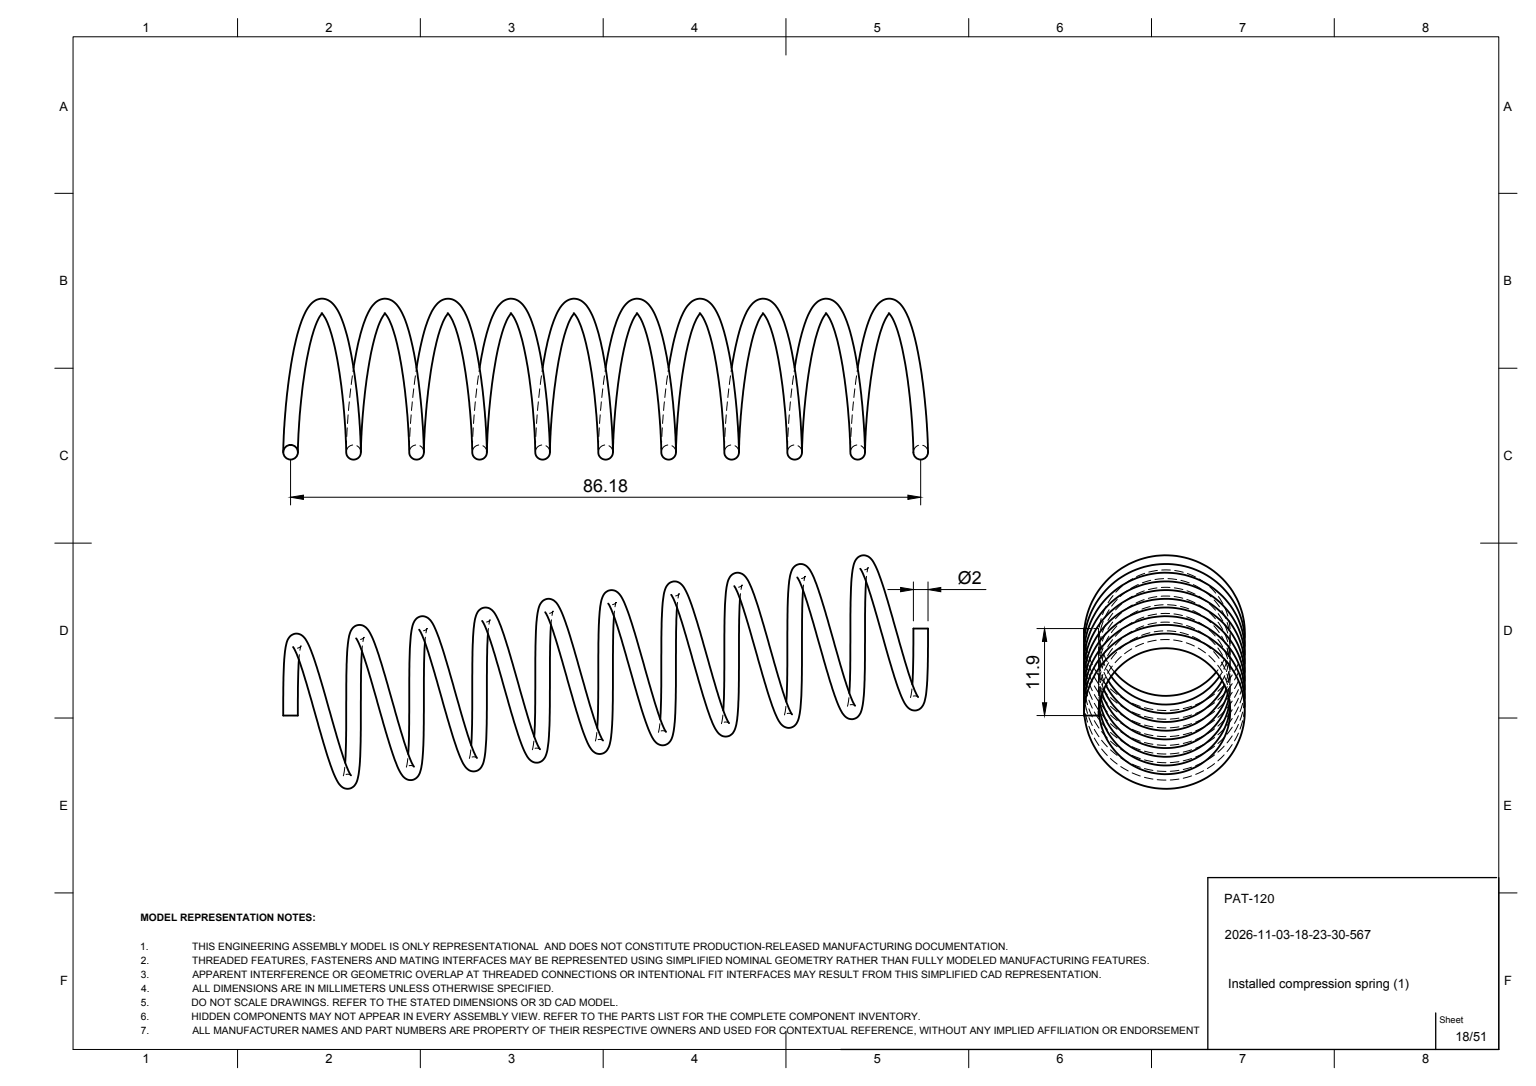
ISO-10303-21;
HEADER;
/* Generated by software containing ST-Developer
 * from STEP Tools, Inc. (www.steptools.com) 
 */

FILE_DESCRIPTION(
/* description */ ('Vibration shaker table dummy'),
/* implementation_level */ '2;1');

FILE_NAME(
/* name */ 'Installed compression spring (1).step',
/* time_stamp */ '2026-10-27T10:55:14-07:00',
/* author */ (''),
/* organization */ (''),
/* preprocessor_version */ 'ST-DEVELOPER v20.2',
/* originating_system */ 'Autodesk Translation Framework v15.17.0.0',
/* authorisation */ '');

FILE_SCHEMA (('AUTOMOTIVE_DESIGN { 1 0 10303 214 3 1 1 }'));
ENDSEC;

DATA;
#10=MECHANICAL_DESIGN_GEOMETRIC_PRESENTATION_REPRESENTATION('',(#699),#22394);
#587=B_SPLINE_CURVE_WITH_KNOTS('',3,(#17470,#17471,#17472,#17473,#17474,
#17475,#17476,#17477,#17478,#17479,#17480,#17481,#17482,#17483,#17484,#17485,
#17486,#17487,#17488,#17489,#17490,#17491,#17492,#17493,#17494,#17495,#17496,
#17497,#17498,#17499,#17500,#17501,#17502,#17503,#17504,#17505,#17506,#17507,
#17508,#17509,#17510,#17511,#17512,#17513,#17514,#17515,#17516,#17517,#17518,
#17519,#17520,#17521,#17522,#17523,#17524,#17525,#17526,#17527,#17528,#17529,
#17530,#17531,#17532,#17533,#17534,#17535,#17536,#17537,#17538,#17539,#17540,
#17541,#17542,#17543,#17544,#17545,#17546,#17547,#17548,#17549,#17550,#17551,
#17552,#17553,#17554,#17555,#17556,#17557,#17558,#17559,#17560,#17561,#17562,
#17563,#17564,#17565,#17566,#17567,#17568,#17569,#17570,#17571,#17572,#17573,
#17574,#17575,#17576,#17577,#17578,#17579,#17580,#17581,#17582,#17583,#17584,
#17585,#17586,#17587,#17588,#17589,#17590,#17591,#17592,#17593,#17594,#17595,
#17596),.UNSPECIFIED.,.F.,.F.,(4,1,1,1,1,1,1,1,1,1,1,1,1,1,1,1,1,1,1,1,
1,1,1,1,1,1,1,1,1,1,1,1,1,1,1,1,1,1,1,1,1,1,1,1,1,1,1,1,1,1,1,1,1,1,1,1,
1,1,1,1,1,1,1,1,1,1,1,1,1,1,1,1,1,1,1,1,1,1,1,1,1,1,1,1,1,1,1,1,1,1,1,1,
1,1,1,1,1,1,1,1,1,1,1,1,1,1,1,1,1,1,1,1,1,1,1,1,1,1,1,1,1,1,1,1,4),(0.,
0.00892857142857143,0.0178571428571429,0.0267857142857143,0.0357142857142857,
0.0446428571428571,0.0535714285714286,0.0625,0.0714285714285714,0.0803571428571428,
0.0892857142857143,0.0982142857142857,0.107142857142857,0.116071428571429,
0.125,0.133928571428571,0.142857142857143,0.150793650793651,0.158730158730159,
0.166666666666667,0.174603174603175,0.182539682539683,0.19047619047619,
0.196428571428571,0.202380952380952,0.208333333333333,0.214285714285714,
0.222222222222222,0.23015873015873,0.238095238095238,0.244047619047619,
0.25,0.261904761904762,0.273809523809524,0.285714285714286,0.297619047619048,
0.30952380952381,0.321428571428571,0.333333333333333,0.337301587301587,
0.341269841269841,0.349206349206349,0.357142857142857,0.365079365079365,
0.373015873015873,0.380952380952381,0.386904761904762,0.392857142857143,
0.404761904761905,0.410714285714286,0.416666666666667,0.422619047619048,
0.428571428571429,0.4375,0.446428571428571,0.455357142857143,0.459821428571429,
0.464285714285714,0.470238095238095,0.476190476190476,0.482142857142857,
0.491071428571429,0.5,0.508928571428571,0.517857142857143,0.526785714285714,
0.535714285714286,0.544642857142857,0.553571428571429,0.5625,0.571428571428571,
0.580357142857143,0.589285714285714,0.598214285714286,0.607142857142857,
0.616071428571429,0.625,0.633928571428571,0.642857142857143,0.650793650793651,
0.658730158730159,0.666666666666667,0.672619047619048,0.678571428571428,
0.684523809523809,0.69047619047619,0.696428571428571,0.702380952380952,
0.708333333333333,0.714285714285714,0.720238095238095,0.726190476190476,
0.732142857142857,0.738095238095238,0.744047619047619,0.75,0.755952380952381,
0.761904761904762,0.76984126984127,0.777777777777778,0.785714285714286,
0.794642857142857,0.803571428571428,0.8125,0.821428571428571,0.830357142857143,
0.839285714285714,0.848214285714286,0.857142857142857,0.866071428571429,
0.875,0.883928571428571,0.892857142857143,0.901785714285714,0.910714285714286,
0.919642857142857,0.928571428571429,0.9375,0.946428571428571,0.955357142857143,
0.964285714285714,0.973214285714286,0.982142857142857,0.991071428571429,
1.),.UNSPECIFIED.);
#591=B_SPLINE_SURFACE_WITH_KNOTS('',3,3,((#16197,#16198,#16199,#16200,#16201,
#16202,#16203,#16204,#16205,#16206,#16207,#16208,#16209,#16210,#16211,#16212,
#16213,#16214,#16215,#16216,#16217,#16218,#16219,#16220,#16221,#16222,#16223,
#16224,#16225,#16226,#16227,#16228,#16229,#16230,#16231,#16232,#16233,#16234,
#16235,#16236,#16237,#16238,#16239,#16240,#16241,#16242,#16243,#16244,#16245,
#16246,#16247,#16248,#16249,#16250,#16251,#16252,#16253,#16254,#16255,#16256,
#16257,#16258,#16259,#16260,#16261,#16262,#16263,#16264,#16265,#16266,#16267,
#16268,#16269,#16270,#16271,#16272,#16273,#16274,#16275,#16276,#16277,#16278,
#16279,#16280,#16281,#16282,#16283,#16284,#16285,#16286,#16287,#16288,#16289,
#16290,#16291,#16292,#16293,#16294,#16295,#16296,#16297,#16298,#16299,#16300,
#16301,#16302,#16303,#16304,#16305,#16306,#16307,#16308,#16309,#16310,#16311,
#16312,#16313,#16314,#16315,#16316,#16317,#16318,#16319,#16320,#16321,#16322,
#16323),(#16324,#16325,#16326,#16327,#16328,#16329,#16330,#16331,#16332,
#16333,#16334,#16335,#16336,#16337,#16338,#16339,#16340,#16341,#16342,#16343,
#16344,#16345,#16346,#16347,#16348,#16349,#16350,#16351,#16352,#16353,#16354,
#16355,#16356,#16357,#16358,#16359,#16360,#16361,#16362,#16363,#16364,#16365,
#16366,#16367,#16368,#16369,#16370,#16371,#16372,#16373,#16374,#16375,#16376,
#16377,#16378,#16379,#16380,#16381,#16382,#16383,#16384,#16385,#16386,#16387,
#16388,#16389,#16390,#16391,#16392,#16393,#16394,#16395,#16396,#16397,#16398,
#16399,#16400,#16401,#16402,#16403,#16404,#16405,#16406,#16407,#16408,#16409,
#16410,#16411,#16412,#16413,#16414,#16415,#16416,#16417,#16418,#16419,#16420,
#16421,#16422,#16423,#16424,#16425,#16426,#16427,#16428,#16429,#16430,#16431,
#16432,#16433,#16434,#16435,#16436,#16437,#16438,#16439,#16440,#16441,#16442,
#16443,#16444,#16445,#16446,#16447,#16448,#16449,#16450),(#16451,#16452,
#16453,#16454,#16455,#16456,#16457,#16458,#16459,#16460,#16461,#16462,#16463,
#16464,#16465,#16466,#16467,#16468,#16469,#16470,#16471,#16472,#16473,#16474,
#16475,#16476,#16477,#16478,#16479,#16480,#16481,#16482,#16483,#16484,#16485,
#16486,#16487,#16488,#16489,#16490,#16491,#16492,#16493,#16494,#16495,#16496,
#16497,#16498,#16499,#16500,#16501,#16502,#16503,#16504,#16505,#16506,#16507,
#16508,#16509,#16510,#16511,#16512,#16513,#16514,#16515,#16516,#16517,#16518,
#16519,#16520,#16521,#16522,#16523,#16524,#16525,#16526,#16527,#16528,#16529,
#16530,#16531,#16532,#16533,#16534,#16535,#16536,#16537,#16538,#16539,#16540,
#16541,#16542,#16543,#16544,#16545,#16546,#16547,#16548,#16549,#16550,#16551,
#16552,#16553,#16554,#16555,#16556,#16557,#16558,#16559,#16560,#16561,#16562,
#16563,#16564,#16565,#16566,#16567,#16568,#16569,#16570,#16571,#16572,#16573,
#16574,#16575,#16576,#16577),(#16578,#16579,#16580,#16581,#16582,#16583,
#16584,#16585,#16586,#16587,#16588,#16589,#16590,#16591,#16592,#16593,#16594,
#16595,#16596,#16597,#16598,#16599,#16600,#16601,#16602,#16603,#16604,#16605,
#16606,#16607,#16608,#16609,#16610,#16611,#16612,#16613,#16614,#16615,#16616,
#16617,#16618,#16619,#16620,#16621,#16622,#16623,#16624,#16625,#16626,#16627,
#16628,#16629,#16630,#16631,#16632,#16633,#16634,#16635,#16636,#16637,#16638,
#16639,#16640,#16641,#16642,#16643,#16644,#16645,#16646,#16647,#16648,#16649,
#16650,#16651,#16652,#16653,#16654,#16655,#16656,#16657,#16658,#16659,#16660,
#16661,#16662,#16663,#16664,#16665,#16666,#16667,#16668,#16669,#16670,#16671,
#16672,#16673,#16674,#16675,#16676,#16677,#16678,#16679,#16680,#16681,#16682,
#16683,#16684,#16685,#16686,#16687,#16688,#16689,#16690,#16691,#16692,#16693,
#16694,#16695,#16696,#16697,#16698,#16699,#16700,#16701,#16702,#16703,#16704),
(#16705,#16706,#16707,#16708,#16709,#16710,#16711,#16712,#16713,#16714,
#16715,#16716,#16717,#16718,#16719,#16720,#16721,#16722,#16723,#16724,#16725,
#16726,#16727,#16728,#16729,#16730,#16731,#16732,#16733,#16734,#16735,#16736,
#16737,#16738,#16739,#16740,#16741,#16742,#16743,#16744,#16745,#16746,#16747,
#16748,#16749,#16750,#16751,#16752,#16753,#16754,#16755,#16756,#16757,#16758,
#16759,#16760,#16761,#16762,#16763,#16764,#16765,#16766,#16767,#16768,#16769,
#16770,#16771,#16772,#16773,#16774,#16775,#16776,#16777,#16778,#16779,#16780,
#16781,#16782,#16783,#16784,#16785,#16786,#16787,#16788,#16789,#16790,#16791,
#16792,#16793,#16794,#16795,#16796,#16797,#16798,#16799,#16800,#16801,#16802,
#16803,#16804,#16805,#16806,#16807,#16808,#16809,#16810,#16811,#16812,#16813,
#16814,#16815,#16816,#16817,#16818,#16819,#16820,#16821,#16822,#16823,#16824,
#16825,#16826,#16827,#16828,#16829,#16830,#16831),(#16832,#16833,#16834,
#16835,#16836,#16837,#16838,#16839,#16840,#16841,#16842,#16843,#16844,#16845,
#16846,#16847,#16848,#16849,#16850,#16851,#16852,#16853,#16854,#16855,#16856,
#16857,#16858,#16859,#16860,#16861,#16862,#16863,#16864,#16865,#16866,#16867,
#16868,#16869,#16870,#16871,#16872,#16873,#16874,#16875,#16876,#16877,#16878,
#16879,#16880,#16881,#16882,#16883,#16884,#16885,#16886,#16887,#16888,#16889,
#16890,#16891,#16892,#16893,#16894,#16895,#16896,#16897,#16898,#16899,#16900,
#16901,#16902,#16903,#16904,#16905,#16906,#16907,#16908,#16909,#16910,#16911,
#16912,#16913,#16914,#16915,#16916,#16917,#16918,#16919,#16920,#16921,#16922,
#16923,#16924,#16925,#16926,#16927,#16928,#16929,#16930,#16931,#16932,#16933,
#16934,#16935,#16936,#16937,#16938,#16939,#16940,#16941,#16942,#16943,#16944,
#16945,#16946,#16947,#16948,#16949,#16950,#16951,#16952,#16953,#16954,#16955,
#16956,#16957,#16958),(#16959,#16960,#16961,#16962,#16963,#16964,#16965,
#16966,#16967,#16968,#16969,#16970,#16971,#16972,#16973,#16974,#16975,#16976,
#16977,#16978,#16979,#16980,#16981,#16982,#16983,#16984,#16985,#16986,#16987,
#16988,#16989,#16990,#16991,#16992,#16993,#16994,#16995,#16996,#16997,#16998,
#16999,#17000,#17001,#17002,#17003,#17004,#17005,#17006,#17007,#17008,#17009,
#17010,#17011,#17012,#17013,#17014,#17015,#17016,#17017,#17018,#17019,#17020,
#17021,#17022,#17023,#17024,#17025,#17026,#17027,#17028,#17029,#17030,#17031,
#17032,#17033,#17034,#17035,#17036,#17037,#17038,#17039,#17040,#17041,#17042,
#17043,#17044,#17045,#17046,#17047,#17048,#17049,#17050,#17051,#17052,#17053,
#17054,#17055,#17056,#17057,#17058,#17059,#17060,#17061,#17062,#17063,#17064,
#17065,#17066,#17067,#17068,#17069,#17070,#17071,#17072,#17073,#17074,#17075,
#17076,#17077,#17078,#17079,#17080,#17081,#17082,#17083,#17084,#17085),
(#17086,#17087,#17088,#17089,#17090,#17091,#17092,#17093,#17094,#17095,
#17096,#17097,#17098,#17099,#17100,#17101,#17102,#17103,#17104,#17105,#17106,
#17107,#17108,#17109,#17110,#17111,#17112,#17113,#17114,#17115,#17116,#17117,
#17118,#17119,#17120,#17121,#17122,#17123,#17124,#17125,#17126,#17127,#17128,
#17129,#17130,#17131,#17132,#17133,#17134,#17135,#17136,#17137,#17138,#17139,
#17140,#17141,#17142,#17143,#17144,#17145,#17146,#17147,#17148,#17149,#17150,
#17151,#17152,#17153,#17154,#17155,#17156,#17157,#17158,#17159,#17160,#17161,
#17162,#17163,#17164,#17165,#17166,#17167,#17168,#17169,#17170,#17171,#17172,
#17173,#17174,#17175,#17176,#17177,#17178,#17179,#17180,#17181,#17182,#17183,
#17184,#17185,#17186,#17187,#17188,#17189,#17190,#17191,#17192,#17193,#17194,
#17195,#17196,#17197,#17198,#17199,#17200,#17201,#17202,#17203,#17204,#17205,
#17206,#17207,#17208,#17209,#17210,#17211,#17212),(#17213,#17214,#17215,
#17216,#17217,#17218,#17219,#17220,#17221,#17222,#17223,#17224,#17225,#17226,
#17227,#17228,#17229,#17230,#17231,#17232,#17233,#17234,#17235,#17236,#17237,
#17238,#17239,#17240,#17241,#17242,#17243,#17244,#17245,#17246,#17247,#17248,
#17249,#17250,#17251,#17252,#17253,#17254,#17255,#17256,#17257,#17258,#17259,
#17260,#17261,#17262,#17263,#17264,#17265,#17266,#17267,#17268,#17269,#17270,
#17271,#17272,#17273,#17274,#17275,#17276,#17277,#17278,#17279,#17280,#17281,
#17282,#17283,#17284,#17285,#17286,#17287,#17288,#17289,#17290,#17291,#17292,
#17293,#17294,#17295,#17296,#17297,#17298,#17299,#17300,#17301,#17302,#17303,
#17304,#17305,#17306,#17307,#17308,#17309,#17310,#17311,#17312,#17313,#17314,
#17315,#17316,#17317,#17318,#17319,#17320,#17321,#17322,#17323,#17324,#17325,
#17326,#17327,#17328,#17329,#17330,#17331,#17332,#17333,#17334,#17335,#17336,
#17337,#17338,#17339),(#17340,#17341,#17342,#17343,#17344,#17345,#17346,
#17347,#17348,#17349,#17350,#17351,#17352,#17353,#17354,#17355,#17356,#17357,
#17358,#17359,#17360,#17361,#17362,#17363,#17364,#17365,#17366,#17367,#17368,
#17369,#17370,#17371,#17372,#17373,#17374,#17375,#17376,#17377,#17378,#17379,
#17380,#17381,#17382,#17383,#17384,#17385,#17386,#17387,#17388,#17389,#17390,
#17391,#17392,#17393,#17394,#17395,#17396,#17397,#17398,#17399,#17400,#17401,
#17402,#17403,#17404,#17405,#17406,#17407,#17408,#17409,#17410,#17411,#17412,
#17413,#17414,#17415,#17416,#17417,#17418,#17419,#17420,#17421,#17422,#17423,
#17424,#17425,#17426,#17427,#17428,#17429,#17430,#17431,#17432,#17433,#17434,
#17435,#17436,#17437,#17438,#17439,#17440,#17441,#17442,#17443,#17444,#17445,
#17446,#17447,#17448,#17449,#17450,#17451,#17452,#17453,#17454,#17455,#17456,
#17457,#17458,#17459,#17460,#17461,#17462,#17463,#17464,#17465,#17466)),
 .UNSPECIFIED.,.T.,.F.,.F.,(4,1,1,1,1,1,1,4),(4,1,1,1,1,1,1,1,1,1,1,1,1,
1,1,1,1,1,1,1,1,1,1,1,1,1,1,1,1,1,1,1,1,1,1,1,1,1,1,1,1,1,1,1,1,1,1,1,1,
1,1,1,1,1,1,1,1,1,1,1,1,1,1,1,1,1,1,1,1,1,1,1,1,1,1,1,1,1,1,1,1,1,1,1,1,
1,1,1,1,1,1,1,1,1,1,1,1,1,1,1,1,1,1,1,1,1,1,1,1,1,1,1,1,1,1,1,1,1,1,1,1,
1,1,1,4),(-3.14159265358979,-2.24399475256414,-1.34639685153848,-0.448798950512828,
0.448798950512828,1.34639685153848,2.24399475256414,3.14159265358979),(0.,
0.00892857142857143,0.0178571428571429,0.0267857142857143,0.0357142857142857,
0.0446428571428571,0.0535714285714286,0.0625,0.0714285714285714,0.0803571428571428,
0.0892857142857143,0.0982142857142857,0.107142857142857,0.116071428571429,
0.125,0.133928571428571,0.142857142857143,0.150793650793651,0.158730158730159,
0.166666666666667,0.174603174603175,0.182539682539683,0.19047619047619,
0.196428571428571,0.202380952380952,0.208333333333333,0.214285714285714,
0.222222222222222,0.23015873015873,0.238095238095238,0.244047619047619,
0.25,0.261904761904762,0.273809523809524,0.285714285714286,0.297619047619048,
0.30952380952381,0.321428571428571,0.333333333333333,0.337301587301587,
0.341269841269841,0.349206349206349,0.357142857142857,0.365079365079365,
0.373015873015873,0.380952380952381,0.386904761904762,0.392857142857143,
0.404761904761905,0.410714285714286,0.416666666666667,0.422619047619048,
0.428571428571429,0.4375,0.446428571428571,0.455357142857143,0.459821428571429,
0.464285714285714,0.470238095238095,0.476190476190476,0.482142857142857,
0.491071428571429,0.5,0.508928571428571,0.517857142857143,0.526785714285714,
0.535714285714286,0.544642857142857,0.553571428571429,0.5625,0.571428571428571,
0.580357142857143,0.589285714285714,0.598214285714286,0.607142857142857,
0.616071428571429,0.625,0.633928571428571,0.642857142857143,0.650793650793651,
0.658730158730159,0.666666666666667,0.672619047619048,0.678571428571428,
0.684523809523809,0.69047619047619,0.696428571428571,0.702380952380952,
0.708333333333333,0.714285714285714,0.720238095238095,0.726190476190476,
0.732142857142857,0.738095238095238,0.744047619047619,0.75,0.755952380952381,
0.761904761904762,0.76984126984127,0.777777777777778,0.785714285714286,
0.794642857142857,0.803571428571428,0.8125,0.821428571428571,0.830357142857143,
0.839285714285714,0.848214285714286,0.857142857142857,0.866071428571429,
0.875,0.883928571428571,0.892857142857143,0.901785714285714,0.910714285714286,
0.919642857142857,0.928571428571429,0.9375,0.946428571428571,0.955357142857143,
0.964285714285714,0.973214285714286,0.982142857142857,0.991071428571429,
1.),.UNSPECIFIED.);
#607=SHAPE_REPRESENTATION_RELATIONSHIP('SRR','None',#22653,#653);
#653=ADVANCED_BREP_SHAPE_REPRESENTATION('',(#745),#22359);
#699=STYLED_ITEM('',(#22961),#745);
#745=MANIFOLD_SOLID_BREP('Body1',#9217);
#1146=PLANE('',#10078);
#1147=PLANE('',#10079);
#1496=FACE_OUTER_BOUND('',#2110,.T.);
#1497=FACE_OUTER_BOUND('',#2111,.T.);
#1498=FACE_OUTER_BOUND('',#2112,.T.);
#2110=EDGE_LOOP('',(#6972,#6973,#6974,#6975));
#2111=EDGE_LOOP('',(#6976));
#2112=EDGE_LOOP('',(#6977));
#4006=CIRCLE('',#10076,0.1);
#4007=CIRCLE('',#10077,0.1);
#4609=VERTEX_POINT('',#17467);
#4610=VERTEX_POINT('',#17469);
#5479=EDGE_CURVE('',#4609,#4609,#4006,.T.);
#5480=EDGE_CURVE('',#4609,#4610,#587,.T.);
#5481=EDGE_CURVE('',#4610,#4610,#4007,.T.);
#6972=ORIENTED_EDGE('',*,*,#5479,.T.);
#6973=ORIENTED_EDGE('',*,*,#5480,.T.);
#6974=ORIENTED_EDGE('',*,*,#5481,.F.);
#6975=ORIENTED_EDGE('',*,*,#5480,.F.);
#6976=ORIENTED_EDGE('',*,*,#5481,.T.);
#6977=ORIENTED_EDGE('',*,*,#5479,.F.);
#8861=ADVANCED_FACE('',(#1496),#591,.T.);
#8862=ADVANCED_FACE('',(#1497),#1146,.T.);
#8863=ADVANCED_FACE('',(#1498),#1147,.F.);
#9217=CLOSED_SHELL('',(#8861,#8862,#8863));
#10075=AXIS2_PLACEMENT_3D('',#16196,#11796,#11797);
#10076=AXIS2_PLACEMENT_3D('',#17468,#11798,#11799);
#10077=AXIS2_PLACEMENT_3D('',#17597,#11800,#11801);
#10078=AXIS2_PLACEMENT_3D('',#17598,#11802,#11803);
#10079=AXIS2_PLACEMENT_3D('',#17599,#11804,#11805);
#11796=DIRECTION('axis',(0.,0.,1.));
#11797=DIRECTION('refdir',(1.,0.,0.));
#11798=DIRECTION('center_axis',(-0.000133356290794322,0.990604928516086,
0.136754735990165));
#11799=DIRECTION('ref_axis',(1.84100680806489E-5,-0.136754734750974,0.990604937492369));
#11800=DIRECTION('center_axis',(0.000133356202123069,0.990604928495684,
0.13675473613804));
#11801=DIRECTION('ref_axis',(-0.722226697925981,0.0946826990341326,-0.685145081939983));
#11802=DIRECTION('center_axis',(0.000133356202123069,0.990604928495684,
0.13675473613804));
#11803=DIRECTION('ref_axis',(-0.722226697925981,0.0946826990341325,-0.685145081939983));
#11804=DIRECTION('center_axis',(-0.000133356290794322,0.990604928516086,
0.136754735990165));
#11805=DIRECTION('ref_axis',(1.84100680806489E-5,-0.136754734750974,0.990604937492369));
#16196=CARTESIAN_POINT('',(0.,0.,0.));
#16197=CARTESIAN_POINT('Ctrl Pts',(-5.00000184100681,4.0136754734751,2.60093950625076));
#16198=CARTESIAN_POINT('Ctrl Pts',(-5.00002711936209,4.20144961727963,2.62686205390075));
#16199=CARTESIAN_POINT('Ctrl Pts',(-5.1076914443916,4.57620101292901,2.67882571929646));
#16200=CARTESIAN_POINT('Ctrl Pts',(-5.54731085839696,4.97011855968613,2.75738770095752));
#16201=CARTESIAN_POINT('Ctrl Pts',(-6.13330829028169,5.07009398433603,2.83651804650349));
#16202=CARTESIAN_POINT('Ctrl Pts',(-6.68676060294283,4.84148936906199,2.91622569034364));
#16203=CARTESIAN_POINT('Ctrl Pts',(-7.03617542740839,4.34995411926946,2.99649057036664));
#16204=CARTESIAN_POINT('Ctrl Pts',(-7.07077171566156,3.74380977688242,3.07730075350998));
#16205=CARTESIAN_POINT('Ctrl Pts',(-6.77566001133407,3.20870450421941,3.15863603264667));
#16206=CARTESIAN_POINT('Ctrl Pts',(-6.23777975703619,2.91082274760045,3.24047540010177));
#16207=CARTESIAN_POINT('Ctrl Pts',(-5.62027751939497,2.94499359194798,3.32279385402167));
#16208=CARTESIAN_POINT('Ctrl Pts',(-5.1128578559771,3.30444603110391,3.40556404882598));
#16209=CARTESIAN_POINT('Ctrl Pts',(-4.87328209631149,3.88170381609706,3.48875576249667));
#16210=CARTESIAN_POINT('Ctrl Pts',(-4.97806047014568,4.50081578134862,3.57233636795591));
#16211=CARTESIAN_POINT('Ctrl Pts',(-5.39799694068156,4.97124635132397,3.65627091939543));
#16212=CARTESIAN_POINT('Ctrl Pts',(-6.00608186722498,5.1467635917961,3.7405223892875));
#16213=CARTESIAN_POINT('Ctrl Pts',(-6.61648592829516,4.97125245378467,3.82505187703477));
#16214=CARTESIAN_POINT('Ctrl Pts',(-7.02504723026834,4.51407458863333,3.90667930466183));
#16215=CARTESIAN_POINT('Ctrl Pts',(-7.14109507248108,3.93953170138583,3.98533819578826));
#16216=CARTESIAN_POINT('Ctrl Pts',(-6.97515546374893,3.40104443225745,4.06097495793453));
#16217=CARTESIAN_POINT('Ctrl Pts',(-6.57122653386479,3.00706128325563,4.13670514732847));
#16218=CARTESIAN_POINT('Ctrl Pts',(-6.02775857632327,2.85377271371871,4.21249751130402));
#16219=CARTESIAN_POINT('Ctrl Pts',(-5.47693199324532,2.97976879840739,4.28832050275612));
#16220=CARTESIAN_POINT('Ctrl Pts',(-5.08889329636147,3.32248782371839,4.35782394322737));
#16221=CARTESIAN_POINT('Ctrl Pts',(-4.90348334427995,3.74815768282725,4.42098503121462));
#16222=CARTESIAN_POINT('Ctrl Pts',(-4.88777846541416,4.16541417756998,4.47779829335302));
#16223=CARTESIAN_POINT('Ctrl Pts',(-5.02572337488508,4.5591407782775,4.53456660974454));
#16224=CARTESIAN_POINT('Ctrl Pts',(-5.32762081329308,4.91046292297288,4.59757802398128));
#16225=CARTESIAN_POINT('Ctrl Pts',(-5.79769987729577,5.12240617534609,4.6667893141555));
#16226=CARTESIAN_POINT('Ctrl Pts',(-6.35744977854988,5.0800953582818,4.74213609062164));
#16227=CARTESIAN_POINT('Ctrl Pts',(-6.7886388886812,4.80135715932747,4.81103357029135));
#16228=CARTESIAN_POINT('Ctrl Pts',(-7.03217914396847,4.41239214657722,4.87351124701705));
#16229=CARTESIAN_POINT('Ctrl Pts',(-7.13592863330475,3.87207852021905,4.94830807653976));
#16230=CARTESIAN_POINT('Ctrl Pts',(-6.87284718079957,3.20107467373212,5.04144479366485));
#16231=CARTESIAN_POINT('Ctrl Pts',(-6.09623481157017,2.82823992504595,5.15254762809713));
#16232=CARTESIAN_POINT('Ctrl Pts',(-5.27971004197149,3.08146490109176,5.26291010705797));
#16233=CARTESIAN_POINT('Ctrl Pts',(-4.85635349881296,3.81715131471987,5.37246078991772));
#16234=CARTESIAN_POINT('Ctrl Pts',(-5.04487949063783,4.63769677411038,5.48113679376609));
#16235=CARTESIAN_POINT('Ctrl Pts',(-5.73589746055469,5.10693196272956,5.58888446285182));
#16236=CARTESIAN_POINT('Ctrl Pts',(-6.37118793757295,5.00949360744693,5.67193196549858));
#16237=CARTESIAN_POINT('Ctrl Pts',(-6.71254361053678,4.74926813559046,5.73087908447486));
#16238=CARTESIAN_POINT('Ctrl Pts',(-6.92618421314144,4.48213635150675,5.77788659686335));
#16239=CARTESIAN_POINT('Ctrl Pts',(-7.05447791083229,4.06557532936466,5.83636209009091));
#16240=CARTESIAN_POINT('Ctrl Pts',(-6.95088091422359,3.55670409484484,5.90607316301112));
#16241=CARTESIAN_POINT('Ctrl Pts',(-6.61900788359635,3.16160526086392,5.97532164754671));
#16242=CARTESIAN_POINT('Ctrl Pts',(-6.14183402203666,2.97493714351951,6.0441065734333));
#16243=CARTESIAN_POINT('Ctrl Pts',(-5.67880942079896,3.03347123408109,6.10673564359386));
#16244=CARTESIAN_POINT('Ctrl Pts',(-5.32735160410172,3.25520230218429,6.16333652454754));
#16245=CARTESIAN_POINT('Ctrl Pts',(-5.03108251682038,3.65479384285351,6.23091649770626));
#16246=CARTESIAN_POINT('Ctrl Pts',(-4.99209121035488,4.17131828916311,6.29799027327816));
#16247=CARTESIAN_POINT('Ctrl Pts',(-5.22308647377139,4.60388582873653,6.36457330678434));
#16248=CARTESIAN_POINT('Ctrl Pts',(-5.49945070307415,4.84205518395227,6.4142703184249));
#16249=CARTESIAN_POINT('Ctrl Pts',(-5.8429108649416,4.96183684549319,6.46373244635463));
#16250=CARTESIAN_POINT('Ctrl Pts',(-6.26484181971828,4.94625056066266,6.52117144061682));
#16251=CARTESIAN_POINT('Ctrl Pts',(-6.69390577408147,4.70907736638303,6.58644589945804));
#16252=CARTESIAN_POINT('Ctrl Pts',(-6.95873462103172,4.22881797506906,6.65940509116432));
#16253=CARTESIAN_POINT('Ctrl Pts',(-6.93269246532923,3.77588585116234,6.71983222414211));
#16254=CARTESIAN_POINT('Ctrl Pts',(-6.77107468324783,3.46412923688142,6.7679659145118));
#16255=CARTESIAN_POINT('Ctrl Pts',(-6.57079871082626,3.25210408080074,6.80796630929164));
#16256=CARTESIAN_POINT('Ctrl Pts',(-6.28566327773964,3.10148204150563,6.85183024182226));
#16257=CARTESIAN_POINT('Ctrl Pts',(-5.9374350403567,3.06238692304077,6.89952195896654));
#16258=CARTESIAN_POINT('Ctrl Pts',(-5.54350254185785,3.16770824417749,6.95498839067594));
#16259=CARTESIAN_POINT('Ctrl Pts',(-5.18977130243312,3.48372162057587,7.01814871426604));
#16260=CARTESIAN_POINT('Ctrl Pts',(-5.04285761799324,3.99497433346206,7.0889328817521));
#16261=CARTESIAN_POINT('Ctrl Pts',(-5.18978309684873,4.50416337482064,7.15948666242575));
#16262=CARTESIAN_POINT('Ctrl Pts',(-5.58408091231752,4.85632154197909,7.22985222665258));
#16263=CARTESIAN_POINT('Ctrl Pts',(-6.10418851591415,4.94454356395432,7.30007283487924));
#16264=CARTESIAN_POINT('Ctrl Pts',(-6.59084588507658,4.74288104801731,7.37019262264957));
#16265=CARTESIAN_POINT('Ctrl Pts',(-6.89540829263521,4.31357351131412,7.44025632549589));
#16266=CARTESIAN_POINT('Ctrl Pts',(-6.92492923689232,3.78812028153619,7.51030900574892));
#16267=CARTESIAN_POINT('Ctrl Pts',(-6.67028427013333,3.32725098620657,7.58039577698737));
#16268=CARTESIAN_POINT('Ctrl Pts',(-6.20897623341015,3.0721729365591,7.65056157443552));
#16269=CARTESIAN_POINT('Ctrl Pts',(-5.68173783558839,3.10162769981329,7.72085085716389));
#16270=CARTESIAN_POINT('Ctrl Pts',(-5.24992919279951,3.40776503869049,7.79130734597953));
#16271=CARTESIAN_POINT('Ctrl Pts',(-5.0465424843122,3.89815513625059,7.86197377424775));
#16272=CARTESIAN_POINT('Ctrl Pts',(-5.13549244911485,4.42345796985394,7.9328916443029));
#16273=CARTESIAN_POINT('Ctrl Pts',(-5.49174629490197,4.82258141736487,8.00410096577713));
#16274=CARTESIAN_POINT('Ctrl Pts',(-6.00803868168598,4.97171279548103,8.07564000534741));
#16275=CARTESIAN_POINT('Ctrl Pts',(-6.52735154266829,4.82257974695955,8.1475451059773));
#16276=CARTESIAN_POINT('Ctrl Pts',(-6.87597910605558,4.43277936154282,8.2171724616343));
#16277=CARTESIAN_POINT('Ctrl Pts',(-6.97565473561711,3.94102818366579,8.28449961898768));
#16278=CARTESIAN_POINT('Ctrl Pts',(-6.8330580514463,3.47827883486752,8.34949563910535));
#16279=CARTESIAN_POINT('Ctrl Pts',(-6.51380412257741,3.1662390255362,8.40942447363317));
#16280=CARTESIAN_POINT('Ctrl Pts',(-6.13368043091516,3.03340218960474,8.46419547601407));
#16281=CARTESIAN_POINT('Ctrl Pts',(-5.77000963425156,3.04672415558585,8.51371979129401));
#16282=CARTESIAN_POINT('Ctrl Pts',(-5.43474033823938,3.19292650787483,8.56348049163152));
#16283=CARTESIAN_POINT('Ctrl Pts',(-5.17477216956946,3.45264130135924,8.61348288970698));
#16284=CARTESIAN_POINT('Ctrl Pts',(-5.02692180394174,3.79107624660051,8.6637316830418));
#16285=CARTESIAN_POINT('Ctrl Pts',(-5.012872576251,4.16195256384123,8.7142309145088));
#16286=CARTESIAN_POINT('Ctrl Pts',(-5.13590369868626,4.51409239039593,8.76498396821864));
#16287=CARTESIAN_POINT('Ctrl Pts',(-5.38031427946466,4.79836661872066,8.81599356007185));
#16288=CARTESIAN_POINT('Ctrl Pts',(-5.71336668770006,4.97458793379134,8.86726173279411));
#16289=CARTESIAN_POINT('Ctrl Pts',(-6.08968356313292,5.01715924274108,8.918789847283));
#16290=CARTESIAN_POINT('Ctrl Pts',(-6.45738481100365,4.91881570416212,8.9705785818587));
#16291=CARTESIAN_POINT('Ctrl Pts',(-6.76530671813857,4.69177684003305,9.02262792715958));
#16292=CARTESIAN_POINT('Ctrl Pts',(-6.96997065785482,4.36635789720065,9.07493719271063));
#16293=CARTESIAN_POINT('Ctrl Pts',(-7.04206467317586,3.98670152421777,9.12750499448518));
#16294=CARTESIAN_POINT('Ctrl Pts',(-6.96988775131722,3.60530323601265,9.18032928987629));
#16295=CARTESIAN_POINT('Ctrl Pts',(-6.7397150976367,3.23792225540337,9.23930487839808));
#16296=CARTESIAN_POINT('Ctrl Pts',(-6.33166237507248,2.97390330552954,9.30453505300732));
#16297=CARTESIAN_POINT('Ctrl Pts',(-5.79979171434613,2.93396143628525,9.37613052323128));
#16298=CARTESIAN_POINT('Ctrl Pts',(-5.29001663621426,3.16323503239153,9.45115011122364));
#16299=CARTESIAN_POINT('Ctrl Pts',(-4.94825545210904,3.64363042187255,9.52964181259955));
#16300=CARTESIAN_POINT('Ctrl Pts',(-4.91325516498484,4.25878443889604,9.61164803507556));
#16301=CARTESIAN_POINT('Ctrl Pts',(-5.2125378502354,4.80126773521892,9.69412424268727));
#16302=CARTESIAN_POINT('Ctrl Pts',(-5.75754644935023,5.10299443985526,9.77704205666351));
#16303=CARTESIAN_POINT('Ctrl Pts',(-6.38261067907029,5.06829058753974,9.86037045595682));
#16304=CARTESIAN_POINT('Ctrl Pts',(-6.89571009340608,4.70469230712254,9.94407602284259));
#16305=CARTESIAN_POINT('Ctrl Pts',(-7.13766387710299,4.12145232028498,10.0281230888647));
#16306=CARTESIAN_POINT('Ctrl Pts',(-7.03181245317105,3.49664097659948,10.112473958668));
#16307=CARTESIAN_POINT('Ctrl Pts',(-6.60841264630813,3.02246212675956,10.1970891533592));
#16308=CARTESIAN_POINT('Ctrl Pts',(-5.99601006835875,2.8458044826624,10.2819276244449));
#16309=CARTESIAN_POINT('Ctrl Pts',(-5.38219522105592,3.02246199100347,10.3669470032346));
#16310=CARTESIAN_POINT('Ctrl Pts',(-4.95579995827654,3.49941222674329,10.452103831618));
#16311=CARTESIAN_POINT('Ctrl Pts',(-4.84844583817861,4.13081136700949,10.5373538681711));
#16312=CARTESIAN_POINT('Ctrl Pts',(-5.0936581339001,4.72286468788687,10.6226522983686));
#16313=CARTESIAN_POINT('Ctrl Pts',(-5.61632959368519,5.09368411438882,10.7079540155997));
#16314=CARTESIAN_POINT('Ctrl Pts',(-6.25587144748665,5.12951914158568,10.7932138961696));
#16315=CARTESIAN_POINT('Ctrl Pts',(-6.81586867421465,4.81987787722662,10.8783870694892));
#16316=CARTESIAN_POINT('Ctrl Pts',(-7.12478685219004,4.26058878480156,10.9634291596385));
#16317=CARTESIAN_POINT('Ctrl Pts',(-7.08884111245123,3.62399110135786,11.0482965343607));
#16318=CARTESIAN_POINT('Ctrl Pts',(-6.72064073263906,3.10540887765364,11.132946666915));
#16319=CARTESIAN_POINT('Ctrl Pts',(-6.13478909423228,2.86304904084892,11.2173381176655));
#16320=CARTESIAN_POINT('Ctrl Pts',(-5.51202996456676,2.96902046658306,11.3014313460436));
#16321=CARTESIAN_POINT('Ctrl Pts',(-5.04310782052529,3.38875866553956,11.3851878225675));
#16322=CARTESIAN_POINT('Ctrl Pts',(-4.92780437314741,3.78964966219835,11.4407823887586));
#16323=CARTESIAN_POINT('Ctrl Pts',(-4.9277773302074,3.99053173009658,11.468514508194));
#16324=CARTESIAN_POINT('Ctrl Pts',(-5.02992177076988,4.01367144562228,2.60093950625076));
#16325=CARTESIAN_POINT('Ctrl Pts',(-5.02994631566222,4.19599723747468,2.62610989942287));
#16326=CARTESIAN_POINT('Ctrl Pts',(-5.13442851066836,4.55976071314582,2.67654110121348));
#16327=CARTESIAN_POINT('Ctrl Pts',(-5.56134974573439,4.94238891673102,2.75283713624014));
#16328=CARTESIAN_POINT('Ctrl Pts',(-6.13078482073242,5.03959236213032,2.82972340704282));
#16329=CARTESIAN_POINT('Ctrl Pts',(-6.66903413561347,4.81735056602101,2.90723061263203));
#16330=CARTESIAN_POINT('Ctrl Pts',(-7.00920598700227,4.33896215278912,2.98534759690749));
#16331=CARTESIAN_POINT('Ctrl Pts',(-7.04301221179128,3.74836605021756,3.06407673097689));
#16332=CARTESIAN_POINT('Ctrl Pts',(-6.75522621874935,3.22631822149203,3.14340922597416));
#16333=CARTESIAN_POINT('Ctrl Pts',(-6.22990332689924,2.93525379627105,3.22333618102973));
#16334=CARTESIAN_POINT('Ctrl Pts',(-5.62589303937123,2.96854762030363,3.3038436934226));
#16335=CARTESIAN_POINT('Ctrl Pts',(-5.12873293812367,3.32056142076909,3.38491511731131));
#16336=CARTESIAN_POINT('Ctrl Pts',(-4.89352413204627,3.88691142159391,3.46653022944677));
#16337=CARTESIAN_POINT('Ctrl Pts',(-4.99635420577753,4.49544431396499,3.54866559717551));
#16338=CARTESIAN_POINT('Ctrl Pts',(-5.40970980407245,4.95874738227325,3.63129493312566));
#16339=CARTESIAN_POINT('Ctrl Pts',(-6.00949882097458,5.13204615047357,3.7143884170231));
#16340=CARTESIAN_POINT('Ctrl Pts',(-6.61281677753053,4.95875572754106,3.79791482865993));
#16341=CARTESIAN_POINT('Ctrl Pts',(-7.01751948399449,4.50615393741704,3.87872895502972));
#16342=CARTESIAN_POINT('Ctrl Pts',(-7.13278308470979,3.9361700979948,3.95675430685426));
#16343=CARTESIAN_POINT('Ctrl Pts',(-6.96798326611628,3.40093725384173,4.03191363881824));
#16344=CARTESIAN_POINT('Ctrl Pts',(-6.56588437170149,3.0085667161029,4.10730455915348));
#16345=CARTESIAN_POINT('Ctrl Pts',(-6.02380660015569,2.85552547105995,4.1828984645294));
#16346=CARTESIAN_POINT('Ctrl Pts',(-5.47331145361356,2.98131883984841,4.25866237696137));
#16347=CARTESIAN_POINT('Ctrl Pts',(-5.08474990971239,3.32433292134206,4.32823136806072));
#16348=CARTESIAN_POINT('Ctrl Pts',(-4.89877468361185,3.75115510083092,4.39155785124952));
#16349=CARTESIAN_POINT('Ctrl Pts',(-4.88295322239428,4.17012206891284,4.44859648966953));
#16350=CARTESIAN_POINT('Ctrl Pts',(-5.02160607801429,4.56601850940387,4.50566779869827));
#16351=CARTESIAN_POINT('Ctrl Pts',(-5.32551155281313,4.91976278214796,4.56909881469144));
#16352=CARTESIAN_POINT('Ctrl Pts',(-5.79947738774271,5.13357696487596,4.63887974785071));
#16353=CARTESIAN_POINT('Ctrl Pts',(-6.36490413396263,5.09095180204026,4.71498361809831));
#16354=CARTESIAN_POINT('Ctrl Pts',(-6.80123703014098,4.8090092395521,4.78468286989168));
#16355=CARTESIAN_POINT('Ctrl Pts',(-7.04805256548717,4.41489660565433,4.84798445867037));
#16356=CARTESIAN_POINT('Ctrl Pts',(-7.15336810542833,3.86676874930573,4.92386067095593));
#16357=CARTESIAN_POINT('Ctrl Pts',(-6.88627890876445,3.18474879109202,5.01849467324825));
#16358=CARTESIAN_POINT('Ctrl Pts',(-6.09541647887762,2.8046825266247,5.13164475831956));
#16359=CARTESIAN_POINT('Ctrl Pts',(-5.26193150367434,3.06284131663416,5.24427210695287));
#16360=CARTESIAN_POINT('Ctrl Pts',(-4.82877192593564,3.81499627184568,5.35628586566125));
#16361=CARTESIAN_POINT('Ctrl Pts',(-5.02163444704993,4.65554191876049,5.46759432075168));
#16362=CARTESIAN_POINT('Ctrl Pts',(-5.73037873412853,5.13706979243288,5.57811802779472));
#16363=CARTESIAN_POINT('Ctrl Pts',(-6.38289817874058,5.03711333080618,5.66341089394338));
#16364=CARTESIAN_POINT('Ctrl Pts',(-6.73374240825734,4.76966130879657,5.72399486558992));
#16365=CARTESIAN_POINT('Ctrl Pts',(-6.95338553801738,4.49503228262409,5.77232227188337));
#16366=CARTESIAN_POINT('Ctrl Pts',(-7.08535371842541,4.06660437649563,5.8324656844589));
#16367=CARTESIAN_POINT('Ctrl Pts',(-6.9787800468111,3.54300210723951,5.90419387832559));
#16368=CARTESIAN_POINT('Ctrl Pts',(-6.63720229094171,3.13634372816596,5.97547164377769));
#16369=CARTESIAN_POINT('Ctrl Pts',(-6.14599330113866,2.94418081803825,6.04628105868442));
#16370=CARTESIAN_POINT('Ctrl Pts',(-5.66932576801709,3.00445079184052,6.11075987344921));
#16371=CARTESIAN_POINT('Ctrl Pts',(-5.30755364968692,3.23270103855633,6.16902649445036));
#16372=CARTESIAN_POINT('Ctrl Pts',(-5.00263765117448,3.6439734402584,6.23858286226327));
#16373=CARTESIAN_POINT('Ctrl Pts',(-4.96258684153503,4.17541554580903,6.30760221503178));
#16374=CARTESIAN_POINT('Ctrl Pts',(-5.20013468158334,4.62018958382737,6.37607271900513));
#16375=CARTESIAN_POINT('Ctrl Pts',(-5.48418644663696,4.86495819379028,6.42715426330249));
#16376=CARTESIAN_POINT('Ctrl Pts',(-5.83700091859451,4.9879746399462,6.47796786909975));
#16377=CARTESIAN_POINT('Ctrl Pts',(-6.27014034257874,4.97194213569626,6.53693781695984));
#16378=CARTESIAN_POINT('Ctrl Pts',(-6.71018721911195,4.7285936197061,6.60390269044994));
#16379=CARTESIAN_POINT('Ctrl Pts',(-6.98138522201246,4.23654963479205,6.67865416688848));
#16380=CARTESIAN_POINT('Ctrl Pts',(-6.95464690173583,3.77319780008151,6.74048646026498));
#16381=CARTESIAN_POINT('Ctrl Pts',(-6.78949328491717,3.45466900883502,6.78967187976814));
#16382=CARTESIAN_POINT('Ctrl Pts',(-6.5850118543023,3.23821591657109,6.83051374195885));
#16383=CARTESIAN_POINT('Ctrl Pts',(-6.29417399113935,3.08462345483403,6.87525911245552));
#16384=CARTESIAN_POINT('Ctrl Pts',(-5.93944085316177,3.04484104332251,6.9238447927216));
#16385=CARTESIAN_POINT('Ctrl Pts',(-5.5386715025412,3.15204520558907,6.98028087779559));
#16386=CARTESIAN_POINT('Ctrl Pts',(-5.17945713800865,3.4731469683138,7.04445344266399));
#16387=CARTESIAN_POINT('Ctrl Pts',(-5.03071086209505,3.9913909494073,7.11621305131435));
#16388=CARTESIAN_POINT('Ctrl Pts',(-5.17946121358645,4.50630591590623,7.18758305156403));
#16389=CARTESIAN_POINT('Ctrl Pts',(-5.57742202874322,4.86150127118643,7.25859677523868));
#16390=CARTESIAN_POINT('Ctrl Pts',(-6.10098354551583,4.95012810222276,7.32929566337638));
#16391=CARTESIAN_POINT('Ctrl Pts',(-6.58957925866623,4.74746480607253,7.39972028560433));
#16392=CARTESIAN_POINT('Ctrl Pts',(-6.8944894280517,4.3173476510197,7.46991402598767));
#16393=CARTESIAN_POINT('Ctrl Pts',(-6.92380025037139,3.79233840638225,7.5399210681067));
#16394=CARTESIAN_POINT('Ctrl Pts',(-6.66985040219311,3.33310620512573,7.60978691749651));
#16395=CARTESIAN_POINT('Ctrl Pts',(-6.21114448179231,3.07967265445472,7.67955782005308));
#16396=CARTESIAN_POINT('Ctrl Pts',(-5.68826793231562,3.10905933047332,7.74928062518807));
#16397=CARTESIAN_POINT('Ctrl Pts',(-5.261141552189,3.41208503440244,7.81900242496648));
#16398=CARTESIAN_POINT('Ctrl Pts',(-5.06052819537421,3.89621323304842,7.88877035751342));
#16399=CARTESIAN_POINT('Ctrl Pts',(-5.14829035086678,4.41356981880071,7.95863124684226));
#16400=CARTESIAN_POINT('Ctrl Pts',(-5.49854581641565,4.80575214553667,8.02863150014836));
#16401=CARTESIAN_POINT('Ctrl Pts',(-6.00502473115743,4.95190610312972,8.09881641615639));
#16402=CARTESIAN_POINT('Ctrl Pts',(-6.51345932322945,4.80576316983501,8.16923087595341));
#16403=CARTESIAN_POINT('Ctrl Pts',(-6.85415432375228,4.4246714653667,8.23729907446955));
#16404=CARTESIAN_POINT('Ctrl Pts',(-6.95137144677235,3.94466951152941,8.30302428873296));
#16405=CARTESIAN_POINT('Ctrl Pts',(-6.81230057517098,3.49356736760953,8.3663911884946));
#16406=CARTESIAN_POINT('Ctrl Pts',(-6.50136287496873,3.18973077505633,8.42475462689054));
#16407=CARTESIAN_POINT('Ctrl Pts',(-6.13148243931581,3.06049314443402,8.47805277620172));
#16408=CARTESIAN_POINT('Ctrl Pts',(-5.77783212683701,3.07346287095625,8.52621486055624));
#16409=CARTESIAN_POINT('Ctrl Pts',(-5.45198580693692,3.21557058633095,8.57457908914575));
#16410=CARTESIAN_POINT('Ctrl Pts',(-5.19943688818408,3.46788583188274,8.62315687629181));
#16411=CARTESIAN_POINT('Ctrl Pts',(-5.05586062852743,3.7965510614861,8.67195580024494));
#16412=CARTESIAN_POINT('Ctrl Pts',(-5.04222328481417,4.15661669267005,8.72098352740896));
#16413=CARTESIAN_POINT('Ctrl Pts',(-5.16164350612221,4.49842329579526,8.77024741487185));
#16414=CARTESIAN_POINT('Ctrl Pts',(-5.39885118948844,4.77432531232921,8.8197540253094));
#16415=CARTESIAN_POINT('Ctrl Pts',(-5.72207722497841,4.94535456295086,8.86950941823545));
#16416=CARTESIAN_POINT('Ctrl Pts',(-6.08730982890222,4.98668115577665,8.91951882966172));
#16417=CARTESIAN_POINT('Ctrl Pts',(-6.44422838706502,4.89123320476848,8.96978715478432));
#16418=CARTESIAN_POINT('Ctrl Pts',(-6.74318709692094,4.67082128233194,9.02031790895771));
#16419=CARTESIAN_POINT('Ctrl Pts',(-6.94195573549741,4.35480362530798,9.0711154801606));
#16420=CARTESIAN_POINT('Ctrl Pts',(-7.01201283432467,3.98598307867038,9.12218006861651));
#16421=CARTESIAN_POINT('Ctrl Pts',(-6.94188012613974,3.61529685245114,9.17351903268827));
#16422=CARTESIAN_POINT('Ctrl Pts',(-6.71809166093455,3.25805588218288,9.23086040513767));
#16423=CARTESIAN_POINT('Ctrl Pts',(-6.32108019967002,3.00111879623715,9.2943252580824));
#16424=CARTESIAN_POINT('Ctrl Pts',(-5.80311451213473,2.96215959372275,9.36404554260668));
#16425=CARTESIAN_POINT('Ctrl Pts',(-5.30615754527745,3.18558411954849,9.4371657391009));
#16426=CARTESIAN_POINT('Ctrl Pts',(-4.97254369393785,3.65434309192426,9.51375567155646));
#16427=CARTESIAN_POINT('Ctrl Pts',(-4.93821839173336,4.25547436438888,9.59388220685397));
#16428=CARTESIAN_POINT('Ctrl Pts',(-5.23099161991045,4.78642955523378,9.67458401443596));
#16429=CARTESIAN_POINT('Ctrl Pts',(-5.76511389845588,5.0822907248545,9.75584348695941));
#16430=CARTESIAN_POINT('Ctrl Pts',(-6.37878715801708,5.04836955778898,9.83763916239741));
#16431=CARTESIAN_POINT('Ctrl Pts',(-6.88349050368107,4.69091453347305,9.91994670353367));
#16432=CARTESIAN_POINT('Ctrl Pts',(-7.12202289533655,4.11635206946976,10.0027386359648));
#16433=CARTESIAN_POINT('Ctrl Pts',(-7.01770835842206,3.49959201553773,10.0859846739843));
#16434=CARTESIAN_POINT('Ctrl Pts',(-6.59911145402226,3.03052923991246,10.1696518435186));
#16435=CARTESIAN_POINT('Ctrl Pts',(-5.99232502515886,2.85530579088301,10.2537046889382));
#16436=CARTESIAN_POINT('Ctrl Pts',(-5.38282080871405,3.03053423729314,10.3381054733215));
#16437=CARTESIAN_POINT('Ctrl Pts',(-4.95845861169447,3.50493632067857,10.4228143871725));
#16438=CARTESIAN_POINT('Ctrl Pts',(-4.85125090468359,4.13438025305609,10.5077898250386));
#16439=CARTESIAN_POINT('Ctrl Pts',(-5.09604965349032,4.72591478984614,10.5929885853316));
#16440=CARTESIAN_POINT('Ctrl Pts',(-5.61917028494442,5.09727783847887,10.6783661345901));
#16441=CARTESIAN_POINT('Ctrl Pts',(-6.26069397088939,5.13340762884881,10.7638768849291));
#16442=CARTESIAN_POINT('Ctrl Pts',(-6.82366484561828,4.82233127266765,10.8494744508988));
#16443=CARTESIAN_POINT('Ctrl Pts',(-7.1349559890951,4.25912401946948,10.9351119297844));
#16444=CARTESIAN_POINT('Ctrl Pts',(-7.09886085350935,3.61669627448514,11.0207420871626));
#16445=CARTESIAN_POINT('Ctrl Pts',(-6.726725604068,3.09227200005312,11.1063179076048));
#16446=CARTESIAN_POINT('Ctrl Pts',(-6.133342143185,2.84661696752136,11.1917922136962));
#16447=CARTESIAN_POINT('Ctrl Pts',(-5.5013537206857,2.95402140345727,11.2771193583949));
#16448=CARTESIAN_POINT('Ctrl Pts',(-5.02457058054561,3.3805972997307,11.3622524411556));
#16449=CARTESIAN_POINT('Ctrl Pts',(-4.90711056796205,3.78884348322686,11.4188571787799));
#16450=CARTESIAN_POINT('Ctrl Pts',(-4.90708301903907,3.99348412566317,11.4471081759781));
#16451=CARTESIAN_POINT('Ctrl Pts',(-5.08958602369426,4.0097422143856,2.62934334321296));
#16452=CARTESIAN_POINT('Ctrl Pts',(-5.08960909668988,4.18113437775253,2.65300432992655));
#16453=CARTESIAN_POINT('Ctrl Pts',(-5.18776711828874,4.52255313756382,2.70034320530108));
#16454=CARTESIAN_POINT('Ctrl Pts',(-5.58805341822381,4.8812003109688,2.77187303447584));
#16455=CARTESIAN_POINT('Ctrl Pts',(-6.12132268985396,4.97214168542557,2.84387592736578));
#16456=CARTESIAN_POINT('Ctrl Pts',(-6.6250405145593,4.76411472905679,2.9164168420007));
#16457=CARTESIAN_POINT('Ctrl Pts',(-6.94331845840803,4.31649001307946,2.98951192726223));
#16458=CARTESIAN_POINT('Ctrl Pts',(-6.9749746715728,3.76378663165257,3.0631944552253));
#16459=CARTESIAN_POINT('Ctrl Pts',(-6.70554141974671,3.27492468355936,3.13748515856724));
#16460=CARTESIAN_POINT('Ctrl Pts',(-6.21320712736269,3.00204398308599,3.21240526971059));
#16461=CARTESIAN_POINT('Ctrl Pts',(-5.64632516705992,3.03317798544545,3.28797050269457));
#16462=CARTESIAN_POINT('Ctrl Pts',(-5.17886703873242,3.36398699143602,3.36419356941742));
#16463=CARTESIAN_POINT('Ctrl Pts',(-4.95714819986703,3.89741137608331,3.44108294567733));
#16464=CARTESIAN_POINT('Ctrl Pts',(-5.05404278332218,4.47200014127016,3.51864333270601));
#16465=CARTESIAN_POINT('Ctrl Pts',(-5.44517543450279,4.91072858287447,3.59687538820991));
#16466=CARTESIAN_POINT('Ctrl Pts',(-6.01453304619026,5.07548882663536,3.67577584985644));
#16467=CARTESIAN_POINT('Ctrl Pts',(-6.58918617679193,4.91071236126573,3.75533744597375));
#16468=CARTESIAN_POINT('Ctrl Pts',(-6.97612300725113,4.4783911747965,3.83257829696492));
#16469=CARTESIAN_POINT('Ctrl Pts',(-7.08686193880412,3.93191614868384,3.90740355882087));
#16470=CARTESIAN_POINT('Ctrl Pts',(-6.92852875642478,3.4169390798757,3.97972468931771));
#16471=CARTESIAN_POINT('Ctrl Pts',(-6.54051538028299,3.03797533609853,4.05251872066026));
#16472=CARTESIAN_POINT('Ctrl Pts',(-6.01539730498932,2.88947896292994,4.1257687615144));
#16473=CARTESIAN_POINT('Ctrl Pts',(-5.48001097232824,3.01154598872243,4.19945421834644));
#16474=CARTESIAN_POINT('Ctrl Pts',(-5.10055444566604,3.34622164586703,4.2673806582065));
#16475=CARTESIAN_POINT('Ctrl Pts',(-4.91828161075229,3.76422683202926,4.32941580368313));
#16476=CARTESIAN_POINT('Ctrl Pts',(-4.90262739686774,4.17579135181212,4.38545682980996));
#16477=CARTESIAN_POINT('Ctrl Pts',(-5.0391283112046,4.56589122264886,4.44169556923536));
#16478=CARTESIAN_POINT('Ctrl Pts',(-5.33934590988134,4.9155506240904,4.50439033686248));
#16479=CARTESIAN_POINT('Ctrl Pts',(-5.80926478584637,5.12782619455085,4.57360252044762));
#16480=CARTESIAN_POINT('Ctrl Pts',(-6.37226870794527,5.0856772459095,4.64938417920319));
#16481=CARTESIAN_POINT('Ctrl Pts',(-6.80864308647832,4.80403298134512,4.71908085712304));
#16482=CARTESIAN_POINT('Ctrl Pts',(-7.05637578676585,4.40869807983537,4.78259624975845));
#16483=CARTESIAN_POINT('Ctrl Pts',(-7.16251945708551,3.85720809409794,4.85895651065945));
#16484=CARTESIAN_POINT('Ctrl Pts',(-6.89330101557501,3.16750144554567,4.95464513573224));
#16485=CARTESIAN_POINT('Ctrl Pts',(-6.08958867663454,2.78013704678207,5.06971861270507));
#16486=CARTESIAN_POINT('Ctrl Pts',(-5.23690622171536,3.04322519808429,5.1849241565956));
#16487=CARTESIAN_POINT('Ctrl Pts',(-4.7906499640607,3.81626968968653,5.3001367232004));
#16488=CARTESIAN_POINT('Ctrl Pts',(-4.9891869239238,4.68549381513598,5.41523683096681));
#16489=CARTESIAN_POINT('Ctrl Pts',(-5.72520324957272,5.18656740249823,5.53009936850738));
#16490=CARTESIAN_POINT('Ctrl Pts',(-6.40658390717164,5.08278139495824,5.61916700647108));
#16491=CARTESIAN_POINT('Ctrl Pts',(-6.77399210603382,4.80276068245273,5.6826055342916));
#16492=CARTESIAN_POINT('Ctrl Pts',(-7.00431863191779,4.51482589298084,5.73328075670049));
#16493=CARTESIAN_POINT('Ctrl Pts',(-7.14314022697556,4.06470659944838,5.79648179082563));
#16494=CARTESIAN_POINT('Ctrl Pts',(-7.03104691519316,3.51311217241579,5.87204065637758));
#16495=CARTESIAN_POINT('Ctrl Pts',(-6.67051256853736,3.08362473260782,5.94730439870082));
#16496=CARTESIAN_POINT('Ctrl Pts',(-6.15081617223352,2.88016159457978,6.02222877098954));
#16497=CARTESIAN_POINT('Ctrl Pts',(-5.64547668178805,2.94393293449389,6.09058436900044));
#16498=CARTESIAN_POINT('Ctrl Pts',(-5.26137505750651,3.1862109614243,6.15244231007988));
#16499=CARTESIAN_POINT('Ctrl Pts',(-4.93725546476308,3.62326890624268,6.22636752336837));
#16500=CARTESIAN_POINT('Ctrl Pts',(-4.89445496952149,4.18887354325382,6.29982377924026));
#16501=CARTESIAN_POINT('Ctrl Pts',(-5.14750606659487,4.66275895844425,6.37276832116607));
#16502=CARTESIAN_POINT('Ctrl Pts',(-5.45026508223206,4.92367181146985,6.4272143147893));
#16503=CARTESIAN_POINT('Ctrl Pts',(-5.82645426351564,5.05485739564245,6.4813918834484));
#16504=CARTESIAN_POINT('Ctrl Pts',(-6.28837776985666,5.03777053987273,6.54427717518941));
#16505=CARTESIAN_POINT('Ctrl Pts',(-6.75766182533428,4.77825976689007,6.6156816277228));
#16506=CARTESIAN_POINT('Ctrl Pts',(-7.04673661650366,4.25369878009071,6.69536196252822));
#16507=CARTESIAN_POINT('Ctrl Pts',(-7.01819649349061,3.76014401169988,6.76121469346688));
#16508=CARTESIAN_POINT('Ctrl Pts',(-6.842405554421,3.42113769275631,6.8135604237066));
#16509=CARTESIAN_POINT('Ctrl Pts',(-6.62491010422242,3.19092779055807,6.85699614151575));
#16510=CARTESIAN_POINT('Ctrl Pts',(-6.31584603200595,3.02775098386413,6.90453688382949));
#16511=CARTESIAN_POINT('Ctrl Pts',(-5.93934547183213,2.98556935104594,6.95609994689215));
#16512=CARTESIAN_POINT('Ctrl Pts',(-5.51459056401894,3.09925021805699,7.01590972758355));
#16513=CARTESIAN_POINT('Ctrl Pts',(-5.13474500286812,3.43902148798019,7.08377081623812));
#16514=CARTESIAN_POINT('Ctrl Pts',(-4.97805736011716,3.98577375141162,7.15945438099295));
#16515=CARTESIAN_POINT('Ctrl Pts',(-5.13473533545388,4.52718957327834,7.23449048550936));
#16516=CARTESIAN_POINT('Ctrl Pts',(-5.55197906444832,4.89921218790737,7.3088943913826));
#16517=CARTESIAN_POINT('Ctrl Pts',(-6.09862301928659,4.99143129445875,7.38268564523815));
#16518=CARTESIAN_POINT('Ctrl Pts',(-6.606479508496,4.78042080069058,7.4558871749407));
#16519=CARTESIAN_POINT('Ctrl Pts',(-6.92180017614838,4.33501283570147,7.52852551129164));
#16520=CARTESIAN_POINT('Ctrl Pts',(-6.95163025782033,3.79411735553687,7.6006304638527));
#16521=CARTESIAN_POINT('Ctrl Pts',(-6.69096189914452,3.32352522627327,7.67223500680259));
#16522=CARTESIAN_POINT('Ctrl Pts',(-6.22294780648661,3.06539982241649,7.74337508280607));
#16523=CARTESIAN_POINT('Ctrl Pts',(-5.69252682775021,3.09561549920305,7.81408937374553));
#16524=CARTESIAN_POINT('Ctrl Pts',(-5.26180726836289,3.40169439692029,7.88441907963459));
#16525=CARTESIAN_POINT('Ctrl Pts',(-5.06089205454407,3.88763262522401,7.9544076442884));
#16526=CARTESIAN_POINT('Ctrl Pts',(-5.14887297659026,4.40380377780348,8.02410059938868));
#16527=CARTESIAN_POINT('Ctrl Pts',(-5.49673854688707,4.79269430477356,8.09354506403565));
#16528=CARTESIAN_POINT('Ctrl Pts',(-5.9966646045048,4.93653868914869,8.16278992414471));
#16529=CARTESIAN_POINT('Ctrl Pts',(-6.49558078845043,4.79271917633619,8.23188451023252));
#16530=CARTESIAN_POINT('Ctrl Pts',(-6.8279254569334,4.42041712558591,8.29832525414164));
#16531=CARTESIAN_POINT('Ctrl Pts',(-6.92211402946376,3.954003052392,8.3621675915439));
#16532=CARTESIAN_POINT('Ctrl Pts',(-6.78734277050336,3.51770084265875,8.42345982961206));
#16533=CARTESIAN_POINT('Ctrl Pts',(-6.48766560070395,3.225159116655,8.4796752721566));
#16534=CARTESIAN_POINT('Ctrl Pts',(-6.1325704869422,3.10120573789478,8.53083075438161));
#16535=CARTESIAN_POINT('Ctrl Pts',(-5.79405420803016,3.11370858336792,8.57692520937968));
#16536=CARTESIAN_POINT('Ctrl Pts',(-5.4830197479851,3.24945336104646,8.62309331209753));
#16537=CARTESIAN_POINT('Ctrl Pts',(-5.24260300270298,3.48976277901665,8.66934329744669));
#16538=CARTESIAN_POINT('Ctrl Pts',(-5.10629115290446,3.80199725893422,8.71569288439519));
#16539=CARTESIAN_POINT('Ctrl Pts',(-5.09344018251244,4.14326532445679,8.76215618077292));
#16540=CARTESIAN_POINT('Ctrl Pts',(-5.20645717818496,4.4665333970135,8.80874723494016));
#16541=CARTESIAN_POINT('Ctrl Pts',(-5.43043962688319,4.72695400089958,8.8554796753622));
#16542=CARTESIAN_POINT('Ctrl Pts',(-5.73508248391682,4.88808365887862,8.90236685255007));
#16543=CARTESIAN_POINT('Ctrl Pts',(-6.0787635295149,4.92691816768683,8.9494215505399));
#16544=CARTESIAN_POINT('Ctrl Pts',(-6.41414963576881,4.83717952868894,8.99665644006685));
#16545=CARTESIAN_POINT('Ctrl Pts',(-6.69473020190159,4.6302656773445,9.04408299555505));
#16546=CARTESIAN_POINT('Ctrl Pts',(-6.88108457282113,4.3339202142424,9.09171380309133));
#16547=CARTESIAN_POINT('Ctrl Pts',(-6.94669400638978,3.98835022131002,9.13955729138141));
#16548=CARTESIAN_POINT('Ctrl Pts',(-6.88100497165465,3.64125145641925,9.1876294691536));
#16549=CARTESIAN_POINT('Ctrl Pts',(-6.6715256852485,3.30689107957766,9.24130014970914));
#16550=CARTESIAN_POINT('Ctrl Pts',(-6.3000268370675,3.06648207926289,9.30068636874497));
#16551=CARTESIAN_POINT('Ctrl Pts',(-5.81535571189857,3.03002056087319,9.36592627913045));
#16552=CARTESIAN_POINT('Ctrl Pts',(-5.35018368207742,3.23913151569331,9.43437243532255));
#16553=CARTESIAN_POINT('Ctrl Pts',(-5.03765642187869,3.67816124377273,9.50611601908226));
#16554=CARTESIAN_POINT('Ctrl Pts',(-5.0053771670949,4.2418152892366,9.58125441399916));
#16555=CARTESIAN_POINT('Ctrl Pts',(-5.28018936987031,4.74045258275521,9.65704272269345));
#16556=CARTESIAN_POINT('Ctrl Pts',(-5.78256486548921,5.01890213015692,9.73349228098031));
#16557=CARTESIAN_POINT('Ctrl Pts',(-6.36108012953608,4.98710397324951,9.81061023053686));
#16558=CARTESIAN_POINT('Ctrl Pts',(-6.8381331976359,4.6494838262545,9.88839989633978));
#16559=CARTESIAN_POINT('Ctrl Pts',(-7.06436608081689,4.10514848060083,9.96686058454078));
#16560=CARTESIAN_POINT('Ctrl Pts',(-6.96547905293281,3.51895521040063,10.0459876562616));
#16561=CARTESIAN_POINT('Ctrl Pts',(-6.56657813231277,3.07154766463719,10.1257725281815));
#16562=CARTESIAN_POINT('Ctrl Pts',(-5.98612686164896,2.90361920268451,10.2062027310299));
#16563=CARTESIAN_POINT('Ctrl Pts',(-5.40077082545841,3.07157466204263,10.2872619783505));
#16564=CARTESIAN_POINT('Ctrl Pts',(-4.99146624135684,3.52863915494167,10.3689302600859));
#16565=CARTESIAN_POINT('Ctrl Pts',(-4.88736373815124,4.1377465623043,10.451183968312));
#16566=CARTESIAN_POINT('Ctrl Pts',(-5.12491722559862,4.7127380657226,10.533996050922));
#16567=CARTESIAN_POINT('Ctrl Pts',(-5.63522883559405,5.07547609755517,10.6173360926148));
#16568=CARTESIAN_POINT('Ctrl Pts',(-6.26402278835794,5.11128141209404,10.7011706911434));
#16569=CARTESIAN_POINT('Ctrl Pts',(-6.81848369757312,4.80536147832042,10.7854632420856));
#16570=CARTESIAN_POINT('Ctrl Pts',(-7.12669178520415,4.24855993845081,10.8701750756115));
#16571=CARTESIAN_POINT('Ctrl Pts',(-7.09123147569517,3.61030668173643,10.9552635816668));
#16572=CARTESIAN_POINT('Ctrl Pts',(-6.72016314892057,3.08670479875095,11.0406872412903));
#16573=CARTESIAN_POINT('Ctrl Pts',(-6.12541064922602,2.84004009606229,11.1263951850926));
#16574=CARTESIAN_POINT('Ctrl Pts',(-5.48884100247513,2.94783409228307,11.2123513814334));
#16575=CARTESIAN_POINT('Ctrl Pts',(-5.00621523782245,3.37901620738018,11.2984814193147));
#16576=CARTESIAN_POINT('Ctrl Pts',(-4.88655208754281,3.79388081444679,11.3560322966674));
#16577=CARTESIAN_POINT('Ctrl Pts',(-4.8865240586904,4.00208649884007,11.3847754541186));
#16578=CARTESIAN_POINT('Ctrl Pts',(-5.11146420993595,3.99650690804392,2.72519407923183));
#16579=CARTESIAN_POINT('Ctrl Pts',(-5.11148671135746,4.16365327148895,2.74826892587012));
#16580=CARTESIAN_POINT('Ctrl Pts',(-5.2073387334252,4.4956152654922,2.79432434811692));
#16581=CARTESIAN_POINT('Ctrl Pts',(-5.59391925930553,4.84117169410349,2.86333869253526));
#16582=CARTESIAN_POINT('Ctrl Pts',(-6.10462940586839,4.92774917966529,2.93229835234812));
#16583=CARTESIAN_POINT('Ctrl Pts',(-6.58327176583413,4.7295348578091,3.00126579937436));
#16584=CARTESIAN_POINT('Ctrl Pts',(-6.88337501314833,4.30667247023342,3.07028767211521));
#16585=CARTESIAN_POINT('Ctrl Pts',(-6.91263235581757,3.78818989461597,3.13941738013105));
#16586=CARTESIAN_POINT('Ctrl Pts',(-6.66103458152486,3.33253551407342,3.2087045265732));
#16587=CARTESIAN_POINT('Ctrl Pts',(-6.20424810480219,3.07978627953998,3.27819919985182));
#16588=CARTESIAN_POINT('Ctrl Pts',(-5.68108649297066,3.10885755482802,3.3479496519015));
#16589=CARTESIAN_POINT('Ctrl Pts',(-5.25169620629678,3.41309053471004,3.41800286743285));
#16590=CARTESIAN_POINT('Ctrl Pts',(-5.04894523297885,3.90154084565558,3.48840393446534));
#16591=CARTESIAN_POINT('Ctrl Pts',(-5.13758046630622,4.42589822713349,3.5591959606558));
#16592=CARTESIAN_POINT('Ctrl Pts',(-5.49376253990945,4.82517927832118,3.63041966550646));
#16593=CARTESIAN_POINT('Ctrl Pts',(-6.01110718354508,4.97476701081733,3.70211331753018));
#16594=CARTESIAN_POINT('Ctrl Pts',(-6.53252812358959,4.82518146836992,3.77431221742951));
#16595=CARTESIAN_POINT('Ctrl Pts',(-6.88337346417075,4.43315294513001,3.84435516038971));
#16596=CARTESIAN_POINT('Ctrl Pts',(-6.98379294743255,3.93768269483383,3.91219940932669));
#16597=CARTESIAN_POINT('Ctrl Pts',(-6.84022481108866,3.47058194620396,3.97779629128527));
#16598=CARTESIAN_POINT('Ctrl Pts',(-6.4880568325447,3.12652942453571,4.04387572836497));
#16599=CARTESIAN_POINT('Ctrl Pts',(-6.0108137656867,2.99147239305588,4.11045064738684));
#16600=CARTESIAN_POINT('Ctrl Pts',(-5.5233657853622,3.10248135006783,4.1775341626934));
#16601=CARTESIAN_POINT('Ctrl Pts',(-5.17709342585232,3.40770238602073,4.23950070121029));
#16602=CARTESIAN_POINT('Ctrl Pts',(-5.01036803456119,3.78984364106918,4.29621638746104));
#16603=CARTESIAN_POINT('Ctrl Pts',(-4.99594479901417,4.1668986052098,4.34755687317996));
#16604=CARTESIAN_POINT('Ctrl Pts',(-5.12120361012274,4.52513375382838,4.39919526106358));
#16605=CARTESIAN_POINT('Ctrl Pts',(-5.39746462943087,4.84705650909992,4.45690227955026));
#16606=CARTESIAN_POINT('Ctrl Pts',(-5.83126731307521,5.04326241388392,4.52080469595619));
#16607=CARTESIAN_POINT('Ctrl Pts',(-6.35313532996607,5.00445569370675,4.59104399722636));
#16608=CARTESIAN_POINT('Ctrl Pts',(-6.75942140048203,4.74254821004542,4.65590506236411));
#16609=CARTESIAN_POINT('Ctrl Pts',(-6.99100458315705,4.37323249129891,4.71524509037977));
#16610=CARTESIAN_POINT('Ctrl Pts',(-7.09069411396853,3.85626121037699,4.78683233689444));
#16611=CARTESIAN_POINT('Ctrl Pts',(-6.83782768759017,3.20584888634675,4.87700820439253));
#16612=CARTESIAN_POINT('Ctrl Pts',(-6.07502780938017,2.83677943548265,4.98629119772695));
#16613=CARTESIAN_POINT('Ctrl Pts',(-5.25818762639893,3.08741236761678,5.09658082375559));
#16614=CARTESIAN_POINT('Ctrl Pts',(-4.82609468064246,3.83314196449917,5.20780897949353));
#16615=CARTESIAN_POINT('Ctrl Pts',(-5.01804196964182,4.68005730215182,5.31989208061913));
#16616=CARTESIAN_POINT('Ctrl Pts',(-5.74046220552027,5.17368997930613,5.43274493776054));
#16617=CARTESIAN_POINT('Ctrl Pts',(-6.41624680437255,5.07190602588026,5.52103403340694));
#16618=CARTESIAN_POINT('Ctrl Pts',(-6.78287311853616,4.79260968907092,5.58431543465606));
#16619=CARTESIAN_POINT('Ctrl Pts',(-7.01337901553013,4.50455289260236,5.63501963999642));
#16620=CARTESIAN_POINT('Ctrl Pts',(-7.15327228278993,4.05225837452208,5.69852711648277));
#16621=CARTESIAN_POINT('Ctrl Pts',(-7.04032973210259,3.49436664439344,5.7749325845684));
#16622=CARTESIAN_POINT('Ctrl Pts',(-6.67391452160444,3.05719409604593,5.85147827278331));
#16623=CARTESIAN_POINT('Ctrl Pts',(-6.14222098191702,2.84858797925773,5.92814825015341));
#16624=CARTESIAN_POINT('Ctrl Pts',(-5.62200447541444,2.9138522941561,5.99849597217976));
#16625=CARTESIAN_POINT('Ctrl Pts',(-5.2245261536068,3.16436876909183,6.06248327165541));
#16626=CARTESIAN_POINT('Ctrl Pts',(-4.88759619272133,3.61827656038866,6.13928274630519));
#16627=CARTESIAN_POINT('Ctrl Pts',(-4.84202233602887,4.20949050233905,6.21606350960167));
#16628=CARTESIAN_POINT('Ctrl Pts',(-5.10798876828044,4.70809462301289,6.29277587691175));
#16629=CARTESIAN_POINT('Ctrl Pts',(-5.42758183608149,4.9836863495513,6.35025953668304));
#16630=CARTESIAN_POINT('Ctrl Pts',(-5.82626078871504,5.12287862051017,6.40767598187554));
#16631=CARTESIAN_POINT('Ctrl Pts',(-6.31765994699635,5.10487041721485,6.47456839078133));
#16632=CARTESIAN_POINT('Ctrl Pts',(-6.81927831104067,4.8279461579424,6.55085139917529));
#16633=CARTESIAN_POINT('Ctrl Pts',(-7.13010460728862,4.26483633665069,6.63640932811157));
#16634=CARTESIAN_POINT('Ctrl Pts',(-7.09962536285686,3.73231937891717,6.70744540954714));
#16635=CARTESIAN_POINT('Ctrl Pts',(-6.90939545722011,3.36533955944663,6.76410161696636));
#16636=CARTESIAN_POINT('Ctrl Pts',(-6.67353014454027,3.11562305636599,6.81121005168782));
#16637=CARTESIAN_POINT('Ctrl Pts',(-6.33759434231894,2.93816086346153,6.86288612599481));
#16638=CARTESIAN_POINT('Ctrl Pts',(-5.9273264322903,2.89211004532868,6.91907330779778));
#16639=CARTESIAN_POINT('Ctrl Pts',(-5.46342269576929,3.01616830676018,6.98439039606857));
#16640=CARTESIAN_POINT('Ctrl Pts',(-5.04741643663609,3.38800643932693,7.05868193967993));
#16641=CARTESIAN_POINT('Ctrl Pts',(-4.87524080338402,3.98808878625817,7.1417508284993));
#16642=CARTESIAN_POINT('Ctrl Pts',(-5.04742888902791,4.58361105136446,7.22427616836105));
#16643=CARTESIAN_POINT('Ctrl Pts',(-5.50696177813016,4.99347012310367,7.30623032326481));
#16644=CARTESIAN_POINT('Ctrl Pts',(-6.10965855662746,5.09519407175069,7.38758749089929));
#16645=CARTESIAN_POINT('Ctrl Pts',(-6.66980784530153,4.86245512149429,7.46832609908296));
#16646=CARTESIAN_POINT('Ctrl Pts',(-7.01748273583442,4.37125721649622,7.54842792966416));
#16647=CARTESIAN_POINT('Ctrl Pts',(-7.05025029721227,3.77526621056693,7.6278786796359));
#16648=CARTESIAN_POINT('Ctrl Pts',(-6.76330668666928,3.25754943443463,7.70666784425883));
#16649=CARTESIAN_POINT('Ctrl Pts',(-6.24929824544846,2.97428480937579,7.78478885750138));
#16650=CARTESIAN_POINT('Ctrl Pts',(-5.66840638807499,3.00762386986153,7.86223910969369));
#16651=CARTESIAN_POINT('Ctrl Pts',(-5.19838941912511,3.34199008402616,7.93901995371726));
#16652=CARTESIAN_POINT('Ctrl Pts',(-4.98021840676051,3.87055262696194,8.0151367421138));
#16653=CARTESIAN_POINT('Ctrl Pts',(-5.0758490831127,4.42932105247054,8.09059869048116));
#16654=CARTESIAN_POINT('Ctrl Pts',(-5.45090874168749,4.84797551191977,8.16541907094984));
#16655=CARTESIAN_POINT('Ctrl Pts',(-5.98662713437262,5.00163881878175,8.23961458119776));
#16656=CARTESIAN_POINT('Ctrl Pts',(-6.51778625442196,4.84800086352156,8.31320648177161));
#16657=CARTESIAN_POINT('Ctrl Pts',(-6.86903664765677,4.4537703574742,8.38351367301843));
#16658=CARTESIAN_POINT('Ctrl Pts',(-6.96763730784423,3.96342515041434,8.45063523465213));
#16659=CARTESIAN_POINT('Ctrl Pts',(-6.82651993949993,3.50789653737747,8.5146520381989));
#16660=CARTESIAN_POINT('Ctrl Pts',(-6.51537470064459,3.20468645809038,8.57297673861431));
#16661=CARTESIAN_POINT('Ctrl Pts',(-6.14917583830804,3.07706708341011,8.62573355281478));
#16662=CARTESIAN_POINT('Ctrl Pts',(-5.80197126391332,3.09006782431164,8.6730209151348));
#16663=CARTESIAN_POINT('Ctrl Pts',(-5.48475623204359,3.22870238611783,8.7201215891855));
#16664=CARTESIAN_POINT('Ctrl Pts',(-5.24095954943397,3.47264590303982,8.76705526211315));
#16665=CARTESIAN_POINT('Ctrl Pts',(-5.10358476082081,3.78776518994619,8.81383109437915));
#16666=CARTESIAN_POINT('Ctrl Pts',(-5.09086869503226,4.13021000186943,8.86046253898069));
#16667=CARTESIAN_POINT('Ctrl Pts',(-5.20381253416027,4.45272962356915,8.90696307606029));
#16668=CARTESIAN_POINT('Ctrl Pts',(-5.42621366433013,4.71104091973399,8.95334665880885));
#16669=CARTESIAN_POINT('Ctrl Pts',(-5.72694035497815,4.86990159293225,8.99962743071014));
#16670=CARTESIAN_POINT('Ctrl Pts',(-6.0642778017449,4.9078453605195,9.04582000979757));
#16671=CARTESIAN_POINT('Ctrl Pts',(-6.39163490242547,4.82007995371208,9.09193880682701));
#16672=CARTESIAN_POINT('Ctrl Pts',(-6.66398013382079,4.61903047711367,9.13799939651309));
#16673=CARTESIAN_POINT('Ctrl Pts',(-6.8438526556467,4.33269428655929,9.184015344281));
#16674=CARTESIAN_POINT('Ctrl Pts',(-6.90674694774413,4.00055605675756,9.23000516247249));
#16675=CARTESIAN_POINT('Ctrl Pts',(-6.84379030170675,3.6686848472656,9.27597658179215));
#16676=CARTESIAN_POINT('Ctrl Pts',(-6.64428368612177,3.35056368320241,9.32706296798443));
#16677=CARTESIAN_POINT('Ctrl Pts',(-6.29248775761018,3.12327735296885,9.38328153460815));
#16678=CARTESIAN_POINT('Ctrl Pts',(-5.83641934789406,3.08928669055234,9.44467550183694));
#16679=CARTESIAN_POINT('Ctrl Pts',(-5.40123529858635,3.28526385412951,9.50873870009347));
#16680=CARTESIAN_POINT('Ctrl Pts',(-5.11066538229929,3.6941010991266,9.57552439669237));
#16681=CARTESIAN_POINT('Ctrl Pts',(-5.08114040909863,4.21597232833541,9.64510193793716));
#16682=CARTESIAN_POINT('Ctrl Pts',(-5.33465538188479,4.6753099831835,9.71495139697783));
#16683=CARTESIAN_POINT('Ctrl Pts',(-5.79581996002734,4.93059943387018,9.78511888244445));
#16684=CARTESIAN_POINT('Ctrl Pts',(-6.32483627711044,4.90128596697204,9.8556490605078));
#16685=CARTESIAN_POINT('Ctrl Pts',(-6.75969561822109,4.59329231159124,9.92658419793803));
#16686=CARTESIAN_POINT('Ctrl Pts',(-6.96535793748658,4.09806931552254,9.99796426902674));
#16687=CARTESIAN_POINT('Ctrl Pts',(-6.87545751761248,3.56575269834969,10.0698265663819));
#16688=CARTESIAN_POINT('Ctrl Pts',(-6.51356552579593,3.15993629343994,10.14220553172));
#16689=CARTESIAN_POINT('Ctrl Pts',(-5.98728606474299,3.00768901099732,10.2151325409728));
#16690=CARTESIAN_POINT('Ctrl Pts',(-5.45650233408849,3.1599478008427,10.2886357289696));
#16691=CARTESIAN_POINT('Ctrl Pts',(-5.08505427049296,3.57461637569863,10.3627398332933));
#16692=CARTESIAN_POINT('Ctrl Pts',(-4.99035571726364,4.12795704288266,10.437466010666));
#16693=CARTESIAN_POINT('Ctrl Pts',(-5.20639519921345,4.65131594928899,10.512831779153));
#16694=CARTESIAN_POINT('Ctrl Pts',(-5.67176741775253,4.98236962341372,10.5888508190908));
#16695=CARTESIAN_POINT('Ctrl Pts',(-6.24692306139383,5.01537477896922,10.6655330858597));
#16696=CARTESIAN_POINT('Ctrl Pts',(-6.75589224783495,4.73489188265989,10.7428843299171));
#16697=CARTESIAN_POINT('Ctrl Pts',(-7.04007219825167,4.22219270063654,10.8209070256255));
#16698=CARTESIAN_POINT('Ctrl Pts',(-7.00764788063291,3.63187265532301,10.8995982295234));
#16699=CARTESIAN_POINT('Ctrl Pts',(-6.66325059419008,3.14520426747428,10.9789543736926));
#16700=CARTESIAN_POINT('Ctrl Pts',(-6.10819988711464,2.91453849274314,11.058960661495));
#16701=CARTESIAN_POINT('Ctrl Pts',(-5.51080240970513,3.01525157871369,11.1396149610308));
#16702=CARTESIAN_POINT('Ctrl Pts',(-5.0551220869379,3.42171950959631,11.2208744527486));
#16703=CARTESIAN_POINT('Ctrl Pts',(-4.94129981546046,3.8153290367668,11.2754818329556));
#16704=CARTESIAN_POINT('Ctrl Pts',(-4.94127315000938,4.01340701770439,11.302826843301));
#16705=CARTESIAN_POINT('Ctrl Pts',(-5.04970739996704,3.98586593555859,2.80233389724905));
#16706=CARTESIAN_POINT('Ctrl Pts',(-5.04973139993852,4.16414391474371,2.82694548283125));
#16707=CARTESIAN_POINT('Ctrl Pts',(-5.15207273229177,4.51778429231705,2.87600729424782));
#16708=CARTESIAN_POINT('Ctrl Pts',(-5.56143445144235,4.88296414226877,2.94901032448266));
#16709=CARTESIAN_POINT('Ctrl Pts',(-6.09813035455802,4.97345393073418,3.02146383671977));
#16710=CARTESIAN_POINT('Ctrl Pts',(-6.59717772837509,4.76616692282312,3.0933916160425));
#16711=CARTESIAN_POINT('Ctrl Pts',(-6.90734650210006,4.32810391152191,3.16483090871071));
#16712=CARTESIAN_POINT('Ctrl Pts',(-6.93678565771805,3.79557382692573,3.2358172810944));
#16713=CARTESIAN_POINT('Ctrl Pts',(-6.67992988144025,3.33168204106518,3.30639099867147));
#16714=CARTESIAN_POINT('Ctrl Pts',(-6.21810435684495,3.07685645369217,3.37659383904583));
#16715=CARTESIAN_POINT('Ctrl Pts',(-5.69393812253209,3.10660642536628,3.4464702010732));
#16716=CARTESIAN_POINT('Ctrl Pts',(-5.26762996911266,3.40941101795258,3.5160661735816));
#16717=CARTESIAN_POINT('Ctrl Pts',(-5.06839285544546,3.89098009041129,3.58542962758082));
#16718=CARTESIAN_POINT('Ctrl Pts',(-5.15561189334424,4.4033880452795,3.65460971073016));
#16719=CARTESIAN_POINT('Ctrl Pts',(-5.50139878752267,4.79014597346869,3.72365678087616));
#16720=CARTESIAN_POINT('Ctrl Pts',(-5.99929163750598,4.93352930590794,3.79262165568086));
#16721=CARTESIAN_POINT('Ctrl Pts',(-6.4970686585488,4.79016609531092,3.86155633018706));
#16722=CARTESIAN_POINT('Ctrl Pts',(-6.82936311892864,4.41814025925142,3.92795746104432));
#16723=CARTESIAN_POINT('Ctrl Pts',(-6.92363065152845,3.95125657284996,3.99187048957157));
#16724=CARTESIAN_POINT('Ctrl Pts',(-6.78882509008231,3.51372124013338,4.05331919673356));
#16725=CARTESIAN_POINT('Ctrl Pts',(-6.46039659394628,3.19327537628355,4.1148982207543));
#16726=CARTESIAN_POINT('Ctrl Pts',(-6.01766263256043,3.06825894175095,4.17664315434586));
#16727=CARTESIAN_POINT('Ctrl Pts',(-5.5675895656199,3.17101321438884,4.23858675780122));
#16728=CARTESIAN_POINT('Ctrl Pts',(-5.2492248404407,3.45189468829417,4.29557696959262));
#16729=CARTESIAN_POINT('Ctrl Pts',(-5.09642736304692,3.80234899603894,4.34758087720494));
#16730=CARTESIAN_POINT('Ctrl Pts',(-5.08330770876435,4.14729318609475,4.39454534850842));
#16731=CARTESIAN_POINT('Ctrl Pts',(-5.19772169901104,4.47431107671478,4.441684267873));
#16732=CARTESIAN_POINT('Ctrl Pts',(-5.44952133586914,4.76762287208321,4.49426708034093));
#16733=CARTESIAN_POINT('Ctrl Pts',(-5.84415803931418,4.94600136701132,4.5523911097729));
#16734=CARTESIAN_POINT('Ctrl Pts',(-6.31810385031458,4.91067419089945,4.61618003218375));
#16735=CARTESIAN_POINT('Ctrl Pts',(-6.68665036777128,4.67303306472473,4.67501868351521));
#16736=CARTESIAN_POINT('Ctrl Pts',(-6.89661632842578,4.33816644176502,4.72882134047227));
#16737=CARTESIAN_POINT('Ctrl Pts',(-6.98697202988125,3.86952263883875,4.79371605024056));
#16738=CARTESIAN_POINT('Ctrl Pts',(-6.75778190933801,3.27983692309617,4.87546960451597));
#16739=CARTESIAN_POINT('Ctrl Pts',(-6.06554426147497,2.94465225979484,4.97466219153242));
#16740=CARTESIAN_POINT('Ctrl Pts',(-5.32245651643167,3.17225925098387,5.07498410984188));
#16741=CARTESIAN_POINT('Ctrl Pts',(-4.92778951573427,3.85238246698133,5.17647141255265));
#16742=CARTESIAN_POINT('Ctrl Pts',(-5.10298048742041,4.62825658707493,5.2791449880962));
#16743=CARTESIAN_POINT('Ctrl Pts',(-5.76740082109715,5.08320984683702,5.38301457542082));
#16744=CARTESIAN_POINT('Ctrl Pts',(-6.39288814393051,4.98967356366879,5.46472968699651));
#16745=CARTESIAN_POINT('Ctrl Pts',(-6.73362172606756,4.73018672825182,5.5235334168208));
#16746=CARTESIAN_POINT('Ctrl Pts',(-6.94828598379921,4.46199079666324,5.57074911296363));
#16747=CARTESIAN_POINT('Ctrl Pts',(-7.07921409875927,4.03950241918021,5.63009246753764));
#16748=CARTESIAN_POINT('Ctrl Pts',(-6.9735205483604,3.5158079784997,5.70180655151957));
#16749=CARTESIAN_POINT('Ctrl Pts',(-6.62817002994743,3.10326385951304,5.77401639409909));
#16750=CARTESIAN_POINT('Ctrl Pts',(-6.12427120584258,2.90518634266498,5.84670069278975));
#16751=CARTESIAN_POINT('Ctrl Pts',(-5.62844987755089,2.96705262654286,5.9137529058833));
#16752=CARTESIAN_POINT('Ctrl Pts',(-5.24775397880409,3.20681158618404,5.97503027044029));
#16753=CARTESIAN_POINT('Ctrl Pts',(-4.92361176447729,3.64307030441914,6.04888078550589));
#16754=CARTESIAN_POINT('Ctrl Pts',(-4.8786775738425,4.21508342665461,6.12319606633034));
#16755=CARTESIAN_POINT('Ctrl Pts',(-5.13751318684674,4.70093420047505,6.19792703986058));
#16756=CARTESIAN_POINT('Ctrl Pts',(-5.45008477387499,4.97066958629773,6.25417272725587));
#16757=CARTESIAN_POINT('Ctrl Pts',(-5.84182005939013,5.10763090725229,6.31060530459667));
#16758=CARTESIAN_POINT('Ctrl Pts',(-6.32690143544471,5.09006208723829,6.37664516231843));
#16759=CARTESIAN_POINT('Ctrl Pts',(-6.82513596476563,4.81560943649251,6.45239369084021));
#16760=CARTESIAN_POINT('Ctrl Pts',(-7.13638106409612,4.25305528894405,6.53792591144884));
#16761=CARTESIAN_POINT('Ctrl Pts',(-7.10620757956584,3.71708032928425,6.60943336872173));
#16762=CARTESIAN_POINT('Ctrl Pts',(-6.91387605566801,3.34581492491729,6.66674540205016));
#16763=CARTESIAN_POINT('Ctrl Pts',(-6.67455235910194,3.09232127351564,6.71456126034345));
#16764=CARTESIAN_POINT('Ctrl Pts',(-6.33233370578708,2.91134781627226,6.76722279147881));
#16765=CARTESIAN_POINT('Ctrl Pts',(-5.91245972381307,2.86404826449612,6.82473115868907));
#16766=CARTESIAN_POINT('Ctrl Pts',(-5.43553481296477,2.9913708635829,6.89188065995733));
#16767=CARTESIAN_POINT('Ctrl Pts',(-5.00519657260536,3.37532227919306,6.96868491584719));
#16768=CARTESIAN_POINT('Ctrl Pts',(-4.82552411217367,3.99939259114819,7.0551070900708));
#16769=CARTESIAN_POINT('Ctrl Pts',(-5.00521412307785,4.62290028123384,7.14150024752713));
#16770=CARTESIAN_POINT('Ctrl Pts',(-5.48875025669925,5.05490216838407,7.22781063449205));
#16771=CARTESIAN_POINT('Ctrl Pts',(-6.1269972684323,5.16315762594082,7.31398827930353));
#16772=CARTESIAN_POINT('Ctrl Pts',(-6.72373757857285,4.91575192086015,7.3999824846241));
#16773=CARTESIAN_POINT('Ctrl Pts',(-7.09632491756847,4.39016444565846,7.48574427967905));
#16774=CARTESIAN_POINT('Ctrl Pts',(-7.13200989794504,3.74901013706194,7.57122577023266));
#16775=CARTESIAN_POINT('Ctrl Pts',(-6.82225282779296,3.18930878099883,7.65638085980697));
#16776=CARTESIAN_POINT('Ctrl Pts',(-6.26460829902145,2.88158315511726,7.7411652953409));
#16777=CARTESIAN_POINT('Ctrl Pts',(-5.63181412213981,2.91757758974348,7.82553705211258));
#16778=CARTESIAN_POINT('Ctrl Pts',(-5.11795160772848,3.28278984563098,7.90945653702931));
#16779=CARTESIAN_POINT('Ctrl Pts',(-4.8786033228671,3.86203570830463,7.99288684593522));
#16780=CARTESIAN_POINT('Ctrl Pts',(-4.9834784860068,4.47596055036701,8.07579394079288));
#16781=CARTESIAN_POINT('Ctrl Pts',(-5.39619233550684,4.93686361644705,8.15814693095131));
#16782=CARTESIAN_POINT('Ctrl Pts',(-5.98659329122227,5.10631370816378,8.23991813342875));
#16783=CARTESIAN_POINT('Ctrl Pts',(-6.57245089294751,4.93690501920364,8.32108349554828));
#16784=CARTESIAN_POINT('Ctrl Pts',(-6.95992631722877,4.50201262961247,8.39863923032397));
#16785=CARTESIAN_POINT('Ctrl Pts',(-7.0686214319773,3.96129877129402,8.47264955664533));
#16786=CARTESIAN_POINT('Ctrl Pts',(-6.91307368893838,3.45942867756379,8.54318002431797));
#16787=CARTESIAN_POINT('Ctrl Pts',(-6.57065452508007,3.12585974988192,8.60735189964973));
#16788=CARTESIAN_POINT('Ctrl Pts',(-6.16834178931565,2.9857181819638,8.66530488614999));
#16789=CARTESIAN_POINT('Ctrl Pts',(-5.78753543501327,3.00003230773149,8.71716373843041));
#16790=CARTESIAN_POINT('Ctrl Pts',(-5.4403035260536,3.15186461292756,8.76872364368885));
#16791=CARTESIAN_POINT('Ctrl Pts',(-5.17405053055488,3.41838442867686,8.8199853550893));
#16792=CARTESIAN_POINT('Ctrl Pts',(-5.02443569797404,3.76179608763484,8.87095033478593));
#16793=CARTESIAN_POINT('Ctrl Pts',(-5.01071112624326,4.13394596082485,8.92162060989388));
#16794=CARTESIAN_POINT('Ctrl Pts',(-5.13318588183195,4.48337012347238,8.97199917604928));
#16795=CARTESIAN_POINT('Ctrl Pts',(-5.37347503109835,4.76228741366554,9.02208969182068));
#16796=CARTESIAN_POINT('Ctrl Pts',(-5.69721116839696,4.93316838834119,9.07189665925581));
#16797=CARTESIAN_POINT('Ctrl Pts',(-6.0589731200314,4.9737322857,9.1214252117248));
#16798=CARTESIAN_POINT('Ctrl Pts',(-6.40861121955068,4.8798544518055,9.1706814415999));
#16799=CARTESIAN_POINT('Ctrl Pts',(-6.69823740111901,4.6658728811842,9.2196716693642));
#16800=CARTESIAN_POINT('Ctrl Pts',(-6.88862583552788,4.36251796004086,9.26840400845727));
#16801=CARTESIAN_POINT('Ctrl Pts',(-6.95478616822326,4.01229514034741,9.31688480847724));
#16802=CARTESIAN_POINT('Ctrl Pts',(-6.88856176972145,3.66404742277028,9.36512658585856));
#16803=CARTESIAN_POINT('Ctrl Pts',(-6.68005169721061,3.33191633214502,9.41846778625709));
#16804=CARTESIAN_POINT('Ctrl Pts',(-6.31460669315386,3.09625457845185,9.47682666960199));
#16805=CARTESIAN_POINT('Ctrl Pts',(-5.84434359292178,3.06162099030016,9.54012231568025));
#16806=CARTESIAN_POINT('Ctrl Pts',(-5.39899847593867,3.26265748297777,9.60569442922599));
#16807=CARTESIAN_POINT('Ctrl Pts',(-5.10429076867847,3.67833278879711,9.67352609353735));
#16808=CARTESIAN_POINT('Ctrl Pts',(-5.07516908125756,4.20415060051834,9.74361156651549));
#16809=CARTESIAN_POINT('Ctrl Pts',(-5.3290043949544,4.66278566701131,9.81338623218308));
#16810=CARTESIAN_POINT('Ctrl Pts',(-5.78623808748219,4.91519435249182,9.88289701703703));
#16811=CARTESIAN_POINT('Ctrl Pts',(-6.3060517965798,4.88578370031614,9.95219212118266));
#16812=CARTESIAN_POINT('Ctrl Pts',(-6.72957149563769,4.58509644581646,10.0213211404762));
#16813=CARTESIAN_POINT('Ctrl Pts',(-6.92791848165719,4.10599187307524,10.0903346248714));
#16814=CARTESIAN_POINT('Ctrl Pts',(-6.84110398927473,3.5952641796134,10.1592838512015));
#16815=CARTESIAN_POINT('Ctrl Pts',(-6.49597787726478,3.2090411855636,10.2282204510126));
#16816=CARTESIAN_POINT('Ctrl Pts',(-5.99800352137511,3.06550216277556,10.2971961468308));
#16817=CARTESIAN_POINT('Ctrl Pts',(-5.49932225007621,3.20903924367168,10.3662624291035));
#16818=CARTESIAN_POINT('Ctrl Pts',(-5.15269705665512,3.59664731894394,10.4354702785398));
#16819=CARTESIAN_POINT('Ctrl Pts',(-5.06513063256634,4.11067041794936,10.5048698000626));
#16820=CARTESIAN_POINT('Ctrl Pts',(-5.26510991061431,4.59418295823839,10.5745100007069));
#16821=CARTESIAN_POINT('Ctrl Pts',(-5.69342119822868,4.89848196985741,10.6444384472408));
#16822=CARTESIAN_POINT('Ctrl Pts',(-6.22048565505005,4.92845041025329,10.7147010475278));
#16823=CARTESIAN_POINT('Ctrl Pts',(-6.68521940982778,4.67207850548342,10.7853416191958));
#16824=CARTESIAN_POINT('Ctrl Pts',(-6.9438915773895,4.20500647688942,10.8564020052726));
#16825=CARTESIAN_POINT('Ctrl Pts',(-6.91427609532709,3.66847163030632,10.9279210525427));
#16826=CARTESIAN_POINT('Ctrl Pts',(-6.60163877912294,3.22685146759834,10.9999360420128));
#16827=CARTESIAN_POINT('Ctrl Pts',(-6.0983327490694,3.01775518242327,11.0724787983336));
#16828=CARTESIAN_POINT('Ctrl Pts',(-5.55680569487759,3.10903241001865,11.1455837409093));
#16829=CARTESIAN_POINT('Ctrl Pts',(-5.14359296425941,3.47760759058162,11.2192690442149));
#16830=CARTESIAN_POINT('Ctrl Pts',(-5.04025170604376,3.83468368477443,11.2688070752426));
#16831=CARTESIAN_POINT('Ctrl Pts',(-5.04022747391784,4.01468628666098,11.2936567480204));
#16832=CARTESIAN_POINT('Ctrl Pts',(-4.95040447126516,3.98592256360826,2.80202053804765));
#16833=CARTESIAN_POINT('Ctrl Pts',(-4.95043091003926,4.18231659775015,2.82913307657434));
#16834=CARTESIAN_POINT('Ctrl Pts',(-5.06329226241015,4.57248759339974,2.88326752141538));
#16835=CARTESIAN_POINT('Ctrl Pts',(-5.51486202834107,4.97524472192967,2.96379225597859));
#16836=CARTESIAN_POINT('Ctrl Pts',(-6.10665528742512,5.07498487533097,3.04369205371294));
#16837=CARTESIAN_POINT('Ctrl Pts',(-6.65633239830572,4.84652999270038,3.12292773711241));
#16838=CARTESIAN_POINT('Ctrl Pts',(-6.9973108765322,4.36466637062073,3.20150215875154));
#16839=CARTESIAN_POINT('Ctrl Pts',(-7.02939784011567,3.78028500733267,3.27940500864084));
#16840=CARTESIAN_POINT('Ctrl Pts',(-6.74810299878159,3.2728050208645,3.35663748365564));
#16841=CARTESIAN_POINT('Ctrl Pts',(-6.24433664339929,2.99519254130349,3.43320130422444));
#16842=CARTESIAN_POINT('Ctrl Pts',(-5.67505771277393,3.02785856483236,3.50910363511194));
#16843=CARTESIAN_POINT('Ctrl Pts',(-5.21440091341081,3.35554690775124,3.58435485999818));
#16844=CARTESIAN_POINT('Ctrl Pts',(-5.00051500372563,3.87366133572611,3.65896947953506));
#16845=CARTESIAN_POINT('Ctrl Pts',(-5.09425563285267,4.42157185945799,3.73296568547931));
#16846=CARTESIAN_POINT('Ctrl Pts',(-5.462150310971,4.83229878934543,3.80636524550889));
#16847=CARTESIAN_POINT('Ctrl Pts',(-5.98798150593187,4.98317282253211,3.87919373094752));
#16848=CARTESIAN_POINT('Ctrl Pts',(-6.50969648071242,4.83232792366873,3.95147945989542));
#16849=CARTESIAN_POINT('Ctrl Pts',(-6.85508457642829,4.44480762082077,4.02059709639111));
#16850=CARTESIAN_POINT('Ctrl Pts',(-6.95204190315741,3.96238793059401,4.08663859114721));
#16851=CARTESIAN_POINT('Ctrl Pts',(-6.81334677614592,3.5136697530612,4.14969044049817));
#16852=CARTESIAN_POINT('Ctrl Pts',(-6.47855613316745,3.18760750471201,4.21241950435217));
#16853=CARTESIAN_POINT('Ctrl Pts',(-6.03081518894969,3.06163527614584,4.27485530762707));
#16854=CARTESIAN_POINT('Ctrl Pts',(-5.57924400076306,3.16517210684398,4.33702916331017));
#16855=CARTESIAN_POINT('Ctrl Pts',(-5.26235852783461,3.44527804080697,4.39381651555624));
#16856=CARTESIAN_POINT('Ctrl Pts',(-5.11131528474039,3.79220578079815,4.44529570200474));
#16857=CARTESIAN_POINT('Ctrl Pts',(-5.09857586586284,4.13174734281154,4.4915318677947));
#16858=CARTESIAN_POINT('Ctrl Pts',(-5.21073898163706,4.45182214864689,4.53768640690343));
#16859=CARTESIAN_POINT('Ctrl Pts',(-5.45607191503352,4.73730787660388,4.5888965218401));
#16860=CARTESIAN_POINT('Ctrl Pts',(-5.83811149272645,4.90959852119948,4.64515384022942));
#16861=CARTESIAN_POINT('Ctrl Pts',(-6.2935786023769,4.87526943519902,4.70646656906679));
#16862=CARTESIAN_POINT('Ctrl Pts',(-6.64527957947667,4.64809167136525,4.76265837292092));
#16863=CARTESIAN_POINT('Ctrl Pts',(-6.84450663785382,4.3300747306855,4.81375039303616));
#16864=CARTESIAN_POINT('Ctrl Pts',(-6.92971145133925,3.88705234376868,4.87509302326313));
#16865=CARTESIAN_POINT('Ctrl Pts',(-6.71365998929187,3.33363363074556,4.95188314417723));
#16866=CARTESIAN_POINT('Ctrl Pts',(-6.06835226953183,3.02231338852184,5.04430471261663));
#16867=CARTESIAN_POINT('Ctrl Pts',(-5.38124050124584,3.23368703501002,5.13712614542432));
#16868=CARTESIAN_POINT('Ctrl Pts',(-5.0189980927801,3.85941422069564,5.23045662938603));
#16869=CARTESIAN_POINT('Ctrl Pts',(-5.17987791457587,4.56911666397937,5.32440725702233));
#16870=CARTESIAN_POINT('Ctrl Pts',(-5.78561808497084,4.98333190955499,5.41907560362953));
#16871=CARTESIAN_POINT('Ctrl Pts',(-6.35398858774582,4.89810415389661,5.49334391945794));
#16872=CARTESIAN_POINT('Ctrl Pts',(-6.66324728871676,4.66257986013562,5.54671917380987));
#16873=CARTESIAN_POINT('Ctrl Pts',(-6.85799457461404,4.41925435012529,5.58955592004314));
#16874=CARTESIAN_POINT('Ctrl Pts',(-6.97670080803186,4.03614191365389,5.64337065998053));
#16875=CARTESIAN_POINT('Ctrl Pts',(-6.88088708133519,3.56137269665567,5.7083859866602));
#16876=CARTESIAN_POINT('Ctrl Pts',(-6.56774877139036,3.18724959659898,5.7738673544995));
#16877=CARTESIAN_POINT('Ctrl Pts',(-6.1105137674248,3.00745058984831,5.83982431290547));
#16878=CARTESIAN_POINT('Ctrl Pts',(-5.6600605012146,3.06356690480529,5.90073862619864));
#16879=CARTESIAN_POINT('Ctrl Pts',(-5.31369872683335,3.28164279863364,5.95648275503902));
#16880=CARTESIAN_POINT('Ctrl Pts',(-5.01835072945631,3.67901092443548,6.02376014793761));
#16881=CARTESIAN_POINT('Ctrl Pts',(-4.97697944716172,4.20135318239159,6.09162170691514));
#16882=CARTESIAN_POINT('Ctrl Pts',(-5.21397626606511,4.64650539147114,6.16007680229855));
#16883=CARTESIAN_POINT('Ctrl Pts',(-5.5009097172886,4.89421993891025,6.21171562591074));
#16884=CARTESIAN_POINT('Ctrl Pts',(-5.86142976014365,5.02037373217275,6.2636524977601));
#16885=CARTESIAN_POINT('Ctrl Pts',(-6.30907789606985,5.0042822573264,6.32459304266943));
#16886=CARTESIAN_POINT('Ctrl Pts',(-6.77062818691674,4.75041637394186,6.39473198710031));
#16887=CARTESIAN_POINT('Ctrl Pts',(-7.06056473245011,4.22724802877586,6.47429953400173));
#16888=CARTESIAN_POINT('Ctrl Pts',(-7.03270980954092,3.72610700206045,6.5411448644184));
#16889=CARTESIAN_POINT('Ctrl Pts',(-6.85223257332155,3.37754933099021,6.59494075166314));
#16890=CARTESIAN_POINT('Ctrl Pts',(-6.62701654047639,3.13891117911654,6.63994397935717));
#16891=CARTESIAN_POINT('Ctrl Pts',(-6.30392790977769,2.96790294404537,6.68966570919111));
#16892=CARTESIAN_POINT('Ctrl Pts',(-5.90593173628063,2.92292306099434,6.74417633692474));
#16893=CARTESIAN_POINT('Ctrl Pts',(-5.45202916168621,3.04391154370486,6.80807460735696));
#16894=CARTESIAN_POINT('Ctrl Pts',(-5.04014333934976,3.41076195351744,6.88151530639827));
#16895=CARTESIAN_POINT('Ctrl Pts',(-4.86667543386624,4.01122016423334,6.96467649603348));
#16896=CARTESIAN_POINT('Ctrl Pts',(-5.04017668893253,4.61531134117894,7.0483417461296));
#16897=CARTESIAN_POINT('Ctrl Pts',(-5.51121666827128,5.03693972368687,7.13247718837409));
#16898=CARTESIAN_POINT('Ctrl Pts',(-6.1375489230342,5.14378348705712,7.21704382881911));
#16899=CARTESIAN_POINT('Ctrl Pts',(-6.72743578865273,4.8998792887582,7.30200118857734));
#16900=CARTESIAN_POINT('Ctrl Pts',(-7.09860950001123,4.37735225371753,7.38730600603053));
#16901=CARTESIAN_POINT('Ctrl Pts',(-7.13497166725086,3.73517172118145,7.47291318935821));
#16902=CARTESIAN_POINT('Ctrl Pts',(-6.82312529085993,3.17041778969823,7.55877577981912));
#16903=CARTESIAN_POINT('Ctrl Pts',(-6.25722282340157,2.85743337580234,7.64484533044293));
#16904=CARTESIAN_POINT('Ctrl Pts',(-5.61036515969932,2.89361956155909,7.73107215137484));
#16905=CARTESIAN_POINT('Ctrl Pts',(-5.08128094643061,3.26891729705054,7.81740565235628));
#16906=CARTESIAN_POINT('Ctrl Pts',(-4.83286127115891,3.86858697173099,7.90379456689586));
#16907=CARTESIAN_POINT('Ctrl Pts',(-4.94160324819162,4.50852949806831,7.99018735499102));
#16908=CARTESIAN_POINT('Ctrl Pts',(-5.37398699340618,4.99222544177309,8.0765322795457));
#16909=CARTESIAN_POINT('Ctrl Pts',(-5.99665145214228,5.1714851524102,8.16277826362009));
#16910=CARTESIAN_POINT('Ctrl Pts',(-6.61834156475152,4.99224641940564,8.24887393319591));
#16911=CARTESIAN_POINT('Ctrl Pts',(-7.03199547791655,4.52864873721892,8.33158922193082));
#16912=CARTESIAN_POINT('Ctrl Pts',(-7.1488251274158,3.94914585462493,8.4109047464235));
#16913=CARTESIAN_POINT('Ctrl Pts',(-6.98164895479995,3.4087990013883,8.48682398223609));
#16914=CARTESIAN_POINT('Ctrl Pts',(-6.61173888808033,3.04810158620894,8.55617610415385));
#16915=CARTESIAN_POINT('Ctrl Pts',(-6.17553818377882,2.89603620626052,8.61900861879084));
#16916=CARTESIAN_POINT('Ctrl Pts',(-5.7615552040565,2.91150440845813,8.67538071920882));
#16917=CARTESIAN_POINT('Ctrl Pts',(-5.38311467013871,3.07688868993499,8.73156698509197));
#16918=CARTESIAN_POINT('Ctrl Pts',(-5.0922662130037,3.3679196502838,8.78755020841222));
#16919=CARTESIAN_POINT('Ctrl Pts',(-4.92846880727788,3.74371374224587,8.84332192844384));
#16920=CARTESIAN_POINT('Ctrl Pts',(-4.9133631481404,4.15171775239193,8.89887160517648));
#16921=CARTESIAN_POINT('Ctrl Pts',(-5.04780408497372,4.5354318905722,8.95418932680646));
#16922=CARTESIAN_POINT('Ctrl Pts',(-5.3119896374796,4.84214892034485,9.00926581135202));
#16923=CARTESIAN_POINT('Ctrl Pts',(-5.66834727126242,5.03028402246597,9.06409240744499));
#16924=CARTESIAN_POINT('Ctrl Pts',(-6.06692750227203,5.07499815830979,9.11866109303675));
#16925=CARTESIAN_POINT('Ctrl Pts',(-6.45240069996794,4.97151173183086,9.17296460291645));
#16926=CARTESIAN_POINT('Ctrl Pts',(-6.77183253555119,4.73551241652737,9.22699618339229));
#16927=CARTESIAN_POINT('Ctrl Pts',(-6.98183516864551,4.40089583076875,9.28075020938804));
#16928=CARTESIAN_POINT('Ctrl Pts',(-7.05478648384277,4.01463129097058,9.33422085838521));
#16929=CARTESIAN_POINT('Ctrl Pts',(-6.98175677735204,3.63071267317424,9.38740512368169));
#16930=CARTESIAN_POINT('Ctrl Pts',(-6.75200291169346,3.26481365293951,9.4461747366418));
#16931=CARTESIAN_POINT('Ctrl Pts',(-6.34977481967191,3.0055454880072,9.51040222003417));
#16932=CARTESIAN_POINT('Ctrl Pts',(-5.83313933101808,2.96762824887196,9.57994102223053));
#16933=CARTESIAN_POINT('Ctrl Pts',(-5.34503066427212,3.18815853893367,9.65182587220209));
#16934=CARTESIAN_POINT('Ctrl Pts',(-5.02311880658278,3.64266389743902,9.72597672677365));
#16935=CARTESIAN_POINT('Ctrl Pts',(-4.99172936034754,4.21533123014454,9.80231318452775));
#16936=CARTESIAN_POINT('Ctrl Pts',(-5.26732576584318,4.71252690360499,9.87799134963007));
#16937=CARTESIAN_POINT('Ctrl Pts',(-5.76100357977955,4.98458611226293,9.95302302651522));
#16938=CARTESIAN_POINT('Ctrl Pts',(-6.3190068491534,4.95256557071688,10.0274239141637));
#16939=CARTESIAN_POINT('Ctrl Pts',(-6.77072516836847,4.63126492501222,10.1012133998304));
#16940=CARTESIAN_POINT('Ctrl Pts',(-6.98059479988593,4.12297966487163,10.1744145058383));
#16941=CARTESIAN_POINT('Ctrl Pts',(-6.88861527514656,3.58510760823276,10.2470537379492));
#16942=CARTESIAN_POINT('Ctrl Pts',(-6.52726164092553,3.18157524040098,10.3191609155057));
#16943=CARTESIAN_POINT('Ctrl Pts',(-6.01022182796172,3.03315029786899,10.3907690096979));
#16944=CARTESIAN_POINT('Ctrl Pts',(-5.4968023601685,3.18155424025962,10.4619139431723));
#16945=CARTESIAN_POINT('Ctrl Pts',(-5.14313043812835,3.57795790884971,10.5326343948435));
#16946=CARTESIAN_POINT('Ctrl Pts',(-5.05500749168914,4.09891712657135,10.6029715309616));
#16947=CARTESIAN_POINT('Ctrl Pts',(-5.25653896569849,4.58456546275314,10.6729687966083));
#16948=CARTESIAN_POINT('Ctrl Pts',(-5.68372978741289,4.88731233402227,10.7426716709992));
#16949=CARTESIAN_POINT('Ctrl Pts',(-6.20465835077419,4.91631905101284,10.812127333084));
#16950=CARTESIAN_POINT('Ctrl Pts',(-6.65989782842747,4.66449619813769,10.881384502152));
#16951=CARTESIAN_POINT('Ctrl Pts',(-6.91089426419046,4.21006249945785,10.9504928961986));
#16952=CARTESIAN_POINT('Ctrl Pts',(-6.88175267869527,3.69248340500686,11.0195035760517));
#16953=CARTESIAN_POINT('Ctrl Pts',(-6.58196495981473,3.26995322639814,11.0884671314299));
#16954=CARTESIAN_POINT('Ctrl Pts',(-6.10334225977061,3.07167484940034,11.1574367940911));
#16955=CARTESIAN_POINT('Ctrl Pts',(-5.59216302952149,3.15826911605838,11.2264605290878));
#16956=CARTESIAN_POINT('Ctrl Pts',(-5.2048518796542,3.50438369446588,11.295597623954));
#16957=CARTESIAN_POINT('Ctrl Pts',(-5.10870508884585,3.83722634528264,11.3417783904471));
#16958=CARTESIAN_POINT('Ctrl Pts',(-5.10868252218105,4.00485746418718,11.3649201584465));
#16959=CARTESIAN_POINT('Ctrl Pts',(-4.88818741853785,3.99652273593062,2.7252971556046));
#16960=CARTESIAN_POINT('Ctrl Pts',(-4.88821540189738,4.20439034906722,2.75399364169819));
#16961=CARTESIAN_POINT('Ctrl Pts',(-5.00770776252223,4.61848709275803,2.81144213686048));
#16962=CARTESIAN_POINT('Ctrl Pts',(-5.48915487885715,5.04852472807647,2.89735480549523));
#16963=CARTESIAN_POINT('Ctrl Pts',(-6.12369806164078,5.15592068267386,2.98303844498173));
#16964=CARTESIAN_POINT('Ctrl Pts',(-6.71613277769504,4.91015860270646,3.06841709492191));
#16965=CARTESIAN_POINT('Ctrl Pts',(-7.08548751283229,4.38888817555002,3.15345804613773));
#16966=CARTESIAN_POINT('Ctrl Pts',(-7.12071612532741,3.75390670031193,3.23811206508075));
#16967=CARTESIAN_POINT('Ctrl Pts',(-6.81423130553448,3.20031927366317,3.3223404682825));
#16968=CARTESIAN_POINT('Ctrl Pts',(-6.26324055802468,2.89636854220571,3.40610337940739));
#16969=CARTESIAN_POINT('Ctrl Pts',(-5.63875242508589,2.93197441766651,3.48936530830127));
#16970=CARTESIAN_POINT('Ctrl Pts',(-5.13221521099117,3.29207938503689,3.5720930071804));
#16971=CARTESIAN_POINT('Ctrl Pts',(-4.89655956374553,3.86258499488725,3.65425670745557));
#16972=CARTESIAN_POINT('Ctrl Pts',(-4.99982380419442,4.46664925394718,3.73582979403668));
#16973=CARTESIAN_POINT('Ctrl Pts',(-5.40561838084694,4.91973814590104,3.81678928615132));
#16974=CARTESIAN_POINT('Ctrl Pts',(-5.9856500350465,5.08614766178258,3.89711563403529));
#16975=CARTESIAN_POINT('Ctrl Pts',(-6.56076716216062,4.91979319813564,3.97679340115906));
#16976=CARTESIAN_POINT('Ctrl Pts',(-6.9409727052211,4.49304289155644,4.05288359943196));
#16977=CARTESIAN_POINT('Ctrl Pts',(-7.0474266977491,3.96276824766782,4.1254636569765));
#16978=CARTESIAN_POINT('Ctrl Pts',(-6.89516904973992,3.47063896532368,4.19460852763417));
#16979=CARTESIAN_POINT('Ctrl Pts',(-6.52878828735251,3.11405822440855,4.26322315390038));
#16980=CARTESIAN_POINT('Ctrl Pts',(-6.04039709877883,2.97684772888406,4.33130874407526));
#16981=CARTESIAN_POINT('Ctrl Pts',(-5.54968575410508,3.08960841211022,4.39887085217573));
#16982=CARTESIAN_POINT('Ctrl Pts',(-5.20683217278918,3.39296272348997,4.4603239618053));
#16983=CARTESIAN_POINT('Ctrl Pts',(-5.04409088312426,3.76709009322268,4.51582250927714));
#16984=CARTESIAN_POINT('Ctrl Pts',(-5.0305243603636,4.13190110393602,4.56548944357907));
#16985=CARTESIAN_POINT('Ctrl Pts',(-5.15069769713791,4.47444293139917,4.61488135084323));
#16986=CARTESIAN_POINT('Ctrl Pts',(-5.41235398803535,4.77868251941044,4.66946114941589));
#16987=CARTESIAN_POINT('Ctrl Pts',(-5.81774434138869,4.96115028608965,4.72912551946573));
#16988=CARTESIAN_POINT('Ctrl Pts',(-6.29798908339291,4.92457568437146,4.7937700973787));
#16989=CARTESIAN_POINT('Ctrl Pts',(-6.66628959161195,4.6862428401203,4.85262918959232));
#16990=CARTESIAN_POINT('Ctrl Pts',(-6.87368370032142,4.35485753503782,4.90584693774055));
#16991=CARTESIAN_POINT('Ctrl Pts',(-6.96176859520356,3.89555011703845,4.96941976954074));
#16992=CARTESIAN_POINT('Ctrl Pts',(-6.73846515358594,3.326843384695,5.04835438030133));
#16993=CARTESIAN_POINT('Ctrl Pts',(-6.08127895739378,3.01150227481938,5.14235131269286));
#16994=CARTESIAN_POINT('Ctrl Pts',(-5.39039177875388,3.22564211348055,5.23571232960406));
#16995=CARTESIAN_POINT('Ctrl Pts',(-5.03125804886121,3.84900889572268,5.32855013951349));
#16996=CARTESIAN_POINT('Ctrl Pts',(-5.19102205882783,4.54707913451127,5.42097217416568));
#16997=CARTESIAN_POINT('Ctrl Pts',(-5.78147777628547,4.9490719546746,5.51310246154377));
#16998=CARTESIAN_POINT('Ctrl Pts',(-6.32878590857654,4.86595140024166,5.58461352654982));
#16999=CARTESIAN_POINT('Ctrl Pts',(-6.62464558290292,4.64052456907037,5.63568596143666));
#17000=CARTESIAN_POINT('Ctrl Pts',(-6.8103718607247,4.408377865189,5.67654311110626));
#17001=CARTESIAN_POINT('Ctrl Pts',(-6.9227678104671,4.04462773784672,5.72760988707244));
#17002=CARTESIAN_POINT('Ctrl Pts',(-6.83202830824635,3.59672191844271,5.78895384400341));
#17003=CARTESIAN_POINT('Ctrl Pts',(-6.53801576444373,3.2459465336319,5.85036988114189));
#17004=CARTESIAN_POINT('Ctrl Pts',(-6.1112121268269,3.07843712584833,5.91191700931704));
#17005=CARTESIAN_POINT('Ctrl Pts',(-5.69297293187985,3.13080016207645,5.96847063433825));
#17006=CARTESIAN_POINT('Ctrl Pts',(-5.37267259566663,3.33259486980722,6.02002493947519));
#17007=CARTESIAN_POINT('Ctrl Pts',(-5.10046464604261,3.69910306117481,6.08205340782182));
#17008=CARTESIAN_POINT('Ctrl Pts',(-5.06292696992554,4.17870579852596,6.14434529872556));
#17009=CARTESIAN_POINT('Ctrl Pts',(-5.27983234324091,4.58585156841641,6.20696440567092));
#17010=CARTESIAN_POINT('Ctrl Pts',(-5.54182383632604,4.81195382016382,6.25410377148257));
#17011=CARTESIAN_POINT('Ctrl Pts',(-5.87037176036449,4.92684977784734,6.30142900406298));
#17012=CARTESIAN_POINT('Ctrl Pts',(-6.277665725455,4.912147013297,6.3568740012257));
#17013=CARTESIAN_POINT('Ctrl Pts',(-6.69688147273969,4.68142565956564,6.42058487897177));
#17014=CARTESIAN_POINT('Ctrl Pts',(-6.95983742269703,4.2067575540915,6.4927687132679));
#17015=CARTESIAN_POINT('Ctrl Pts',(-6.93454926747412,3.7524263987416,6.55336958191222));
#17016=CARTESIAN_POINT('Ctrl Pts',(-6.77094221790365,3.43645100527889,6.60213705006757));
#17017=CARTESIAN_POINT('Ctrl Pts',(-6.56675769701475,3.22009853002638,6.64293797584287));
#17018=CARTESIAN_POINT('Ctrl Pts',(-6.27376286057791,3.06500756365233,6.68803045805404));
#17019=CARTESIAN_POINT('Ctrl Pts',(-5.91262828551806,3.02417323682573,6.7374938299492));
#17020=CARTESIAN_POINT('Ctrl Pts',(-5.50041955363556,3.13401397168084,6.79552405315717));
#17021=CARTESIAN_POINT('Ctrl Pts',(-5.12579134765909,3.46752514898312,6.86231607408146));
#17022=CARTESIAN_POINT('Ctrl Pts',(-4.96753625041387,4.0146614836518,6.93810751304089));
#17023=CARTESIAN_POINT('Ctrl Pts',(-5.1258462367197,4.56667432610493,7.01456115074844));
#17024=CARTESIAN_POINT('Ctrl Pts',(-5.55738945542098,4.95330479961627,7.09168401731796));
#17025=CARTESIAN_POINT('Ctrl Pts',(-6.13343345309169,5.0518789878103,7.16947953573716));
#17026=CARTESIAN_POINT('Ctrl Pts',(-6.67830016319192,4.82695811831511,7.24794698514151));
#17027=CARTESIAN_POINT('Ctrl Pts',(-7.02287341594567,4.34252758285008,7.32708173585149));
#17028=CARTESIAN_POINT('Ctrl Pts',(-7.05716836822738,3.74409198272662,7.40687517558502));
#17029=CARTESIAN_POINT('Ctrl Pts',(-6.76546001393813,3.21489650644473,7.48731481614497));
#17030=CARTESIAN_POINT('Ctrl Pts',(-6.23276792464148,2.91974253368875,7.56838433004706));
#17031=CARTESIAN_POINT('Ctrl Pts',(-5.62012631091812,2.95351650439889,7.6500636810307));
#17032=CARTESIAN_POINT('Ctrl Pts',(-5.11578092937486,3.31062596268586,7.73232921118835));
#17033=CARTESIAN_POINT('Ctrl Pts',(-4.87716301346901,3.88521462852368,7.81515385688724));
#17034=CARTESIAN_POINT('Ctrl Pts',(-4.98150003080198,4.50259039415197,7.89850713183724));
#17035=CARTESIAN_POINT('Ctrl Pts',(-5.40084975729399,4.97257222017584,7.98235571360354));
#17036=CARTESIAN_POINT('Ctrl Pts',(-6.00920307899455,5.1483232714495,8.06666278343668));
#17037=CARTESIAN_POINT('Ctrl Pts',(-6.62101815995564,4.97255948752676,8.15139018914161));
#17038=CARTESIAN_POINT('Ctrl Pts',(-7.031197198535,4.5137306423188,8.23334232564202));
#17039=CARTESIAN_POINT('Ctrl Pts',(-7.14810753526542,3.93609131852819,8.31243675863358));
#17040=CARTESIAN_POINT('Ctrl Pts',(-6.98085185281347,3.39401206249462,8.38858984271055));
#17041=CARTESIAN_POINT('Ctrl Pts',(-6.60786439273102,3.0297840906944,8.45858050620251));
#17042=CARTESIAN_POINT('Ctrl Pts',(-6.16543932526409,2.87532757953747,8.5223305258315));
#17043=CARTESIAN_POINT('Ctrl Pts',(-5.74360228126044,2.8909186429676,8.57978397402559));
#17044=CARTESIAN_POINT('Ctrl Pts',(-5.35620785573692,3.06001727071349,8.63729389811813));
#17045=CARTESIAN_POINT('Ctrl Pts',(-5.05708743686595,3.35908200537455,8.69485647369181));
#17046=CARTESIAN_POINT('Ctrl Pts',(-4.88780606075004,3.74701902455501,8.75245114704132));
#17047=CARTESIAN_POINT('Ctrl Pts',(-4.87196989522485,4.1700891625295,8.81006291512397));
#17048=CARTESIAN_POINT('Ctrl Pts',(-5.0118054178791,4.56971615713679,8.8676763948023));
#17049=CARTESIAN_POINT('Ctrl Pts',(-5.28792248480184,4.890542511533,8.92527629977779));
#17050=CARTESIAN_POINT('Ctrl Pts',(-5.66198182516304,5.08820876432408,8.98284725651621));
#17051=CARTESIAN_POINT('Ctrl Pts',(-6.0820877117984,5.13549890117965,9.04037419150282));
#17052=CARTESIAN_POINT('Ctrl Pts',(-6.49000316987433,5.02614937727024,9.09784167889789));
#17053=CARTESIAN_POINT('Ctrl Pts',(-6.82935485126433,4.77562168586658,9.15523548794978));
#17054=CARTESIAN_POINT('Ctrl Pts',(-7.05332363279532,4.41902744506835,9.212539258798));
#17055=CARTESIAN_POINT('Ctrl Pts',(-7.13149777824104,4.0058899312146,9.26974207432468));
#17056=CARTESIAN_POINT('Ctrl Pts',(-7.05325025901744,3.59384616685398,9.32682158392224));
#17057=CARTESIAN_POINT('Ctrl Pts',(-6.80601788545062,3.19983310992077,9.39010187571138));
#17058=CARTESIAN_POINT('Ctrl Pts',(-6.37157118006669,2.91948826298353,9.45950184637294));
#17059=CARTESIAN_POINT('Ctrl Pts',(-5.81129742273106,2.87811150813228,9.53491939436006));
#17060=CARTESIAN_POINT('Ctrl Pts',(-5.28002903323734,3.11786749908228,9.61315039744257));
#17061=CARTESIAN_POINT('Ctrl Pts',(-4.9283350120672,3.6139208970815,9.69411146456086));
#17062=CARTESIAN_POINT('Ctrl Pts',(-4.89370159918598,4.24102415054889,9.77770799761992));
#17063=CARTESIAN_POINT('Ctrl Pts',(-5.19607987629306,4.78697274776535,9.86079177231777));
#17064=CARTESIAN_POINT('Ctrl Pts',(-5.73907951104547,5.08640154454074,9.94333062311419));
#17065=CARTESIAN_POINT('Ctrl Pts',(-6.35384370981652,5.05124052418518,10.0252959393708));
#17066=CARTESIAN_POINT('Ctrl Pts',(-6.85201199676228,4.69698298891633,10.1066623538334));
#17067=CARTESIAN_POINT('Ctrl Pts',(-7.08354537291699,4.13627475394443,10.1874080858196));
#17068=CARTESIAN_POINT('Ctrl Pts',(-6.98206739002019,3.54305655090038,10.2675149918412));
#17069=CARTESIAN_POINT('Ctrl Pts',(-6.58379031327503,3.09841677074597,10.3469687190531));
#17070=CARTESIAN_POINT('Ctrl Pts',(-6.01478263762881,2.93521361028816,10.4257587680015));
#17071=CARTESIAN_POINT('Ctrl Pts',(-5.45099736693054,3.09836839685132,10.5038785653285));
#17072=CARTESIAN_POINT('Ctrl Pts',(-5.06379832767988,3.53270296534894,10.5813254926886));
#17073=CARTESIAN_POINT('Ctrl Pts',(-4.96787158020713,4.10149828156937,10.6581009257139));
#17074=CARTESIAN_POINT('Ctrl Pts',(-5.18734967510211,4.62953051145273,10.7342101718087));
#17075=CARTESIAN_POINT('Ctrl Pts',(-5.65009570631128,4.9570153326714,10.8096625555231));
#17076=CARTESIAN_POINT('Ctrl Pts',(-6.21132939882819,4.98785053970112,10.8844711049253));
#17077=CARTESIAN_POINT('Ctrl Pts',(-6.69884790173685,4.71765887213222,10.9586530325065));
#17078=CARTESIAN_POINT('Ctrl Pts',(-6.96572373527273,4.23348678541994,11.0322283773605));
#17079=CARTESIAN_POINT('Ctrl Pts',(-6.93439113090648,3.68591170270209,11.1052227079854));
#17080=CARTESIAN_POINT('Ctrl Pts',(-6.61898532491596,3.24226468152419,11.177660612388));
#17081=CARTESIAN_POINT('Ctrl Pts',(-6.11957413084598,3.03597618734333,11.2495797434453));
#17082=CARTESIAN_POINT('Ctrl Pts',(-5.59059433608062,3.12614738105264,11.3209988490037));
#17083=CARTESIAN_POINT('Ctrl Pts',(-5.19328964279077,3.48207627459039,11.391988770315));
#17084=CARTESIAN_POINT('Ctrl Pts',(-5.09580204375325,3.8211227121471,11.4389948522726));
#17085=CARTESIAN_POINT('Ctrl Pts',(-5.09577912292024,3.99138468562821,11.4624998143295));
#17086=CARTESIAN_POINT('Ctrl Pts',(-4.91064567402416,4.00976796878862,2.62933128061604));
#17087=CARTESIAN_POINT('Ctrl Pts',(-4.91067314116014,4.21380094025299,2.65749838774693));
#17088=CARTESIAN_POINT('Ctrl Pts',(-5.02777738329904,4.62104843715925,2.71397001944354));
#17089=CARTESIAN_POINT('Ctrl Pts',(-5.50410058883396,5.04740518005545,2.79904516502667));
#17090=CARTESIAN_POINT('Ctrl Pts',(-6.13662098078803,5.15502614256399,2.8844538444374));
#17091=CARTESIAN_POINT('Ctrl Pts',(-6.73153984852692,4.90888416817942,2.97014996728053));
#17092=CARTESIAN_POINT('Ctrl Pts',(-7.10531686090369,4.3823820288213,3.05608627462904));
#17093=CARTESIAN_POINT('Ctrl Pts',(-7.14175290484821,3.73630540538697,3.14221378953781));
#17094=CARTESIAN_POINT('Ctrl Pts',(-6.82832380401177,3.16895406741704,3.2284825451846));
#17095=CARTESIAN_POINT('Ctrl Pts',(-6.26048494912823,2.85504067087679,3.31484168882952));
#17096=CARTESIAN_POINT('Ctrl Pts',(-5.61239401723101,2.8914159142622,3.40123983352415));
#17097=CARTESIAN_POINT('Ctrl Pts',(-5.08310915284364,3.26700614953085,3.48762540366753));
#17098=CARTESIAN_POINT('Ctrl Pts',(-4.83502303080036,3.86619292249913,3.57394686629917));
#17099=CARTESIAN_POINT('Ctrl Pts',(-4.94364485875093,4.50465820699671,3.66015309210022));
#17100=CARTESIAN_POINT('Ctrl Pts',(-5.37453858626572,4.98650442879576,3.74619359342917));
#17101=CARTESIAN_POINT('Ctrl Pts',(-5.99413141917538,5.16474071398009,3.83201900827667));
#17102=CARTESIAN_POINT('Ctrl Pts',(-6.61181106100534,4.98652297157529,3.91758092543883));
#17103=CARTESIAN_POINT('Ctrl Pts',(-7.02227060414855,4.5263763294177,3.99967575252517));
#17104=CARTESIAN_POINT('Ctrl Pts',(-7.13784103488286,3.95201571751744,4.07830186066915));
#17105=CARTESIAN_POINT('Ctrl Pts',(-6.97254187154243,3.41698947452407,4.15347334639407));
#17106=CARTESIAN_POINT('Ctrl Pts',(-6.57314391987666,3.02798986662469,4.22830470821497));
#17107=CARTESIAN_POINT('Ctrl Pts',(-6.03910362822948,2.87777890366138,4.30276940850961));
#17108=CARTESIAN_POINT('Ctrl Pts',(-5.50111638215199,3.00124361271675,4.37684151437551));
#17109=CARTESIAN_POINT('Ctrl Pts',(-5.12440677043376,3.33442645158616,4.44436384283435));
#17110=CARTESIAN_POINT('Ctrl Pts',(-4.94533142154725,3.74599828483902,4.50542710461716));
#17111=CARTESIAN_POINT('Ctrl Pts',(-4.93036487906514,4.14774216402424,4.56013064511645));
#17112=CARTESIAN_POINT('Ctrl Pts',(-5.06278625695976,4.52525542320837,4.61457215171803));
#17113=CARTESIAN_POINT('Ctrl Pts',(-5.35129270421363,4.86073725652708,4.67476507190189));
#17114=CARTESIAN_POINT('Ctrl Pts',(-5.79842815503293,5.06199857300563,4.74058481530442));
#17115=CARTESIAN_POINT('Ctrl Pts',(-6.32805210185099,5.02164378663595,4.81188343610946));
#17116=CARTESIAN_POINT('Ctrl Pts',(-6.73397836813742,4.75890073365287,4.87677640400761));
#17117=CARTESIAN_POINT('Ctrl Pts',(-6.96231833364606,4.39398026117723,4.93538713836827));
#17118=CARTESIAN_POINT('Ctrl Pts',(-7.05915977358153,3.88872695911014,5.00532566139195));
#17119=CARTESIAN_POINT('Ctrl Pts',(-6.81364543951855,3.26450858713251,5.09201750919447));
#17120=CARTESIAN_POINT('Ctrl Pts',(-6.09460099291618,2.92021072923617,5.19484760834442));
#17121=CARTESIAN_POINT('Ctrl Pts',(-5.34288634734843,3.15403642928638,5.29649459932079));
#17122=CARTESIAN_POINT('Ctrl Pts',(-4.95511179166806,3.82898994813764,5.39697466684311));
#17123=CARTESIAN_POINT('Ctrl Pts',(-5.12784877934483,4.5789002529021,5.49632431032147));
#17124=CARTESIAN_POINT('Ctrl Pts',(-5.75808193491375,5.00652139410731,5.59458312904311));
#17125=CARTESIAN_POINT('Ctrl Pts',(-6.33648847978147,4.9176997738217,5.67021042750851));
#17126=CARTESIAN_POINT('Ctrl Pts',(-6.64717042016579,4.68086196158556,5.7238634266878));
#17127=CARTESIAN_POINT('Ctrl Pts',(-6.8416021768888,4.4377454131655,5.7666459073939));
#17128=CARTESIAN_POINT('Ctrl Pts',(-6.95838649841976,4.05859511388473,5.81987849038407));
#17129=CARTESIAN_POINT('Ctrl Pts',(-6.86409262477757,3.59516210271433,5.88336519673482));
#17130=CARTESIAN_POINT('Ctrl Pts',(-6.56159285132325,3.23491908721871,5.94650414310894));
#17131=CARTESIAN_POINT('Ctrl Pts',(-6.12597096392956,3.06439414322808,6.0093074876293));
#17132=CARTESIAN_POINT('Ctrl Pts',(-5.70236686608432,3.1178198313833,6.0666074274623));
#17133=CARTESIAN_POINT('Ctrl Pts',(-5.380122673147,3.32104386243891,6.11850003188511));
#17134=CARTESIAN_POINT('Ctrl Pts',(-5.10787632083129,3.68804825140651,6.18058621464548));
#17135=CARTESIAN_POINT('Ctrl Pts',(-5.07150998975464,4.16419512411157,6.24242799659425));
#17136=CARTESIAN_POINT('Ctrl Pts',(-5.28523589548665,4.56477917688274,6.30407580547538));
#17137=CARTESIAN_POINT('Ctrl Pts',(-5.54182678085649,4.78602928247548,6.35023001525522));
#17138=CARTESIAN_POINT('Ctrl Pts',(-5.86180686221491,4.89774513429516,6.39631824503907));
#17139=CARTESIAN_POINT('Ctrl Pts',(-6.25632381243741,4.88331058519368,6.45002738837586));
#17140=CARTESIAN_POINT('Ctrl Pts',(-6.65956563830335,4.66083856383486,6.51135090062564));
#17141=CARTESIAN_POINT('Ctrl Pts',(-6.91027780675986,4.20716380710425,6.58030861757756));
#17142=CARTESIAN_POINT('Ctrl Pts',(-6.88590244429634,3.77627762225862,6.63779205741682));
#17143=CARTESIAN_POINT('Ctrl Pts',(-6.73144725053243,3.47814458537331,6.68381436763788));
#17144=CARTESIAN_POINT('Ctrl Pts',(-6.53934056134022,3.27467116868115,6.72219376697843));
#17145=CARTESIAN_POINT('Ctrl Pts',(-6.26469099012521,3.12942239607942,6.76445537433218));
#17146=CARTESIAN_POINT('Ctrl Pts',(-5.92756071018149,3.09141899259667,6.81062906476635));
#17147=CARTESIAN_POINT('Ctrl Pts',(-5.54422762795656,3.19370614855236,6.86459746291479));
#17148=CARTESIAN_POINT('Ctrl Pts',(-5.19754383461621,3.50275475425966,6.92643961530437));
#17149=CARTESIAN_POINT('Ctrl Pts',(-5.05200826635028,4.00707808463828,6.99628451388278));
#17150=CARTESIAN_POINT('Ctrl Pts',(-5.19756546451278,4.51362930224783,7.06644704414763));
#17151=CARTESIAN_POINT('Ctrl Pts',(-5.59238323965525,4.86704223287948,7.13697216632295));
#17152=CARTESIAN_POINT('Ctrl Pts',(-6.11767746247401,4.95673943944794,7.20790194100564));
#17153=CARTESIAN_POINT('Ctrl Pts',(-6.61329771063287,4.75199100760384,7.27927638914268));
#17154=CARTESIAN_POINT('Ctrl Pts',(-6.92614139128033,4.31199654687507,7.35113275685342));
#17155=CARTESIAN_POINT('Ctrl Pts',(-6.9571975467719,3.76912800444529,7.423505503059));
#17156=CARTESIAN_POINT('Ctrl Pts',(-6.69270421729341,3.28932324733122,7.49642599103587));
#17157=CARTESIAN_POINT('Ctrl Pts',(-6.20970313639906,3.02166164921741,7.56992237489679));
#17158=CARTESIAN_POINT('Ctrl Pts',(-5.65382074027343,3.05222706591483,7.6440193764838));
#17159=CARTESIAN_POINT('Ctrl Pts',(-5.19557577726472,3.37654361855234,7.71873817781238));
#17160=CARTESIAN_POINT('Ctrl Pts',(-4.97826782350353,3.8993856502534,7.79409623237114));
#17161=CARTESIAN_POINT('Ctrl Pts',(-5.07323032347364,4.46254478708333,7.8701072988587));
#17162=CARTESIAN_POINT('Ctrl Pts',(-5.45660461493641,4.89258443960897,7.94678104764465));
#17163=CARTESIAN_POINT('Ctrl Pts',(-6.01476043904619,5.05413520603182,8.02412366366451));
#17164=CARTESIAN_POINT('Ctrl Pts',(-6.57833417536576,4.89257846081219,8.10213633415574));
#17165=CARTESIAN_POINT('Ctrl Pts',(-6.95791455951021,4.46849196311221,8.17790431988503));
#17166=CARTESIAN_POINT('Ctrl Pts',(-7.06677953585924,3.93210458538223,8.25133598903447));
#17167=CARTESIAN_POINT('Ctrl Pts',(-6.91104997509509,3.42641897107069,8.32235387143313));
#17168=CARTESIAN_POINT('Ctrl Pts',(-6.56180003391545,3.08496284345591,8.38791761690604));
#17169=CARTESIAN_POINT('Ctrl Pts',(-6.1456027543353,2.93950056003664,8.44788090837857));
#17170=CARTESIAN_POINT('Ctrl Pts',(-5.74726494655331,2.95408057114023,8.50212056041012));
#17171=CARTESIAN_POINT('Ctrl Pts',(-5.37997347796744,3.11424831925692,8.55663140495941));
#17172=CARTESIAN_POINT('Ctrl Pts',(-5.09521302131359,3.398741500323,8.61139836356879));
#17173=CARTESIAN_POINT('Ctrl Pts',(-4.93332872853029,3.76934469312497,8.66641734559057));
#17174=CARTESIAN_POINT('Ctrl Pts',(-4.91797985132647,4.17523812948246,8.72167965701057));
#17175=CARTESIAN_POINT('Ctrl Pts',(-5.05255498515063,4.56031052428824,8.77717618865606));
#17176=CARTESIAN_POINT('Ctrl Pts',(-5.31959588340143,4.87083760394284,8.8328971565062));
#17177=CARTESIAN_POINT('Ctrl Pts',(-5.68301975204626,5.06306855289482,8.8888322510767));
#17178=CARTESIAN_POINT('Ctrl Pts',(-6.09304345640864,5.10939106913153,8.9449704650885));
#17179=CARTESIAN_POINT('Ctrl Pts',(-6.49299926542453,5.00234860987632,9.0013005551928));
#17180=CARTESIAN_POINT('Ctrl Pts',(-6.82728558123996,4.75577359118481,9.05781010687818));
#17181=CARTESIAN_POINT('Ctrl Pts',(-7.04898193413433,4.40311250625515,9.11448771824764));
#17182=CARTESIAN_POINT('Ctrl Pts',(-7.12683472133885,3.99261902493127,9.17131822613187));
#17183=CARTESIAN_POINT('Ctrl Pts',(-7.04888849326792,3.58126093676225,9.22829351281217));
#17184=CARTESIAN_POINT('Ctrl Pts',(-6.80115336644072,3.18607404321642,9.29173806496654));
#17185=CARTESIAN_POINT('Ctrl Pts',(-6.36340806671669,2.90314134363089,9.36168982415459));
#17186=CARTESIAN_POINT('Ctrl Pts',(-5.79521809157173,2.86076218208454,9.43817009255432));
#17187=CARTESIAN_POINT('Ctrl Pts',(-5.25303743345012,3.10496561424916,9.51797381367612));
#17188=CARTESIAN_POINT('Ctrl Pts',(-4.89152375820551,3.61390066850146,9.60108189482633));
#17189=CARTESIAN_POINT('Ctrl Pts',(-4.85515441846885,4.26189522592992,9.68745972603124));
#17190=CARTESIAN_POINT('Ctrl Pts',(-5.16913161772041,4.82994539286161,9.77385897203761));
#17191=CARTESIAN_POINT('Ctrl Pts',(-5.73709448115372,5.14376652967341,9.86022814221491));
#17192=CARTESIAN_POINT('Ctrl Pts',(-6.38432934899975,5.10727832815486,9.94651569088689));
#17193=CARTESIAN_POINT('Ctrl Pts',(-6.91211582322222,4.73257940117262,10.0326707058309));
#17194=CARTESIAN_POINT('Ctrl Pts',(-7.15907764199467,4.13576450802929,10.1186429904321));
#17195=CARTESIAN_POINT('Ctrl Pts',(-7.05090943421799,3.50076864306298,10.2043834497604));
#17196=CARTESIAN_POINT('Ctrl Pts',(-6.62285029522974,3.0222538279605,10.2898443693623));
#17197=CARTESIAN_POINT('Ctrl Pts',(-6.00816185318676,2.84554979076536,10.3749796891461));
#17198=CARTESIAN_POINT('Ctrl Pts',(-5.39636640563317,3.02223735184074,10.4597452748207));
#17199=CARTESIAN_POINT('Ctrl Pts',(-4.97444631827297,3.49505631224499,10.5440991603088));
#17200=CARTESIAN_POINT('Ctrl Pts',(-4.86936219074472,4.11653834401228,10.6280018501589));
#17201=CARTESIAN_POINT('Ctrl Pts',(-5.10966657939444,4.69526291176007,10.7114164772727));
#17202=CARTESIAN_POINT('Ctrl Pts',(-5.61786112599645,5.05513200621197,10.7943090970552));
#17203=CARTESIAN_POINT('Ctrl Pts',(-6.23548062728098,5.08919687074565,10.8766487583371));
#17204=CARTESIAN_POINT('Ctrl Pts',(-6.77273351761296,4.79153197079639,10.9584079804219));
#17205=CARTESIAN_POINT('Ctrl Pts',(-7.06706144191725,4.25760734730938,11.0395622358401));
#17206=CARTESIAN_POINT('Ctrl Pts',(-7.03247204506743,3.65362797051252,11.1200915649221));
#17207=CARTESIAN_POINT('Ctrl Pts',(-6.68464073545661,3.16451872129078,11.1999774348503));
#17208=CARTESIAN_POINT('Ctrl Pts',(-6.13448705150615,2.9373955420016,11.2792100819558));
#17209=CARTESIAN_POINT('Ctrl Pts',(-5.55274917991616,3.03673746832776,11.3577723501083));
#17210=CARTESIAN_POINT('Ctrl Pts',(-5.11690626681905,3.42739822280303,11.4356762391777));
#17211=CARTESIAN_POINT('Ctrl Pts',(-5.01030553006867,3.79852727230778,11.4871434418717));
#17212=CARTESIAN_POINT('Ctrl Pts',(-5.01028050391396,3.98442812877985,11.5128073789705));
#17213=CARTESIAN_POINT('Ctrl Pts',(-4.97008191124374,4.01367950132792,2.60093950625076));
#17214=CARTESIAN_POINT('Ctrl Pts',(-4.97010792325056,4.20690339805964,2.62761440178568));
#17215=CARTESIAN_POINT('Ctrl Pts',(-5.08093760858241,4.59266080489006,2.68110100679445));
#17216=CARTESIAN_POINT('Ctrl Pts',(-5.53326658633966,4.99790615693166,2.76192472631994));
#17217=CARTESIAN_POINT('Ctrl Pts',(-6.13586869185039,5.10068577095782,2.84329383983683));
#17218=CARTESIAN_POINT('Ctrl Pts',(-6.7045933205602,4.86571328724988,2.92519942604245));
#17219=CARTESIAN_POINT('Ctrl Pts',(-7.06331496787067,4.36097514622367,3.00761019396623));
#17220=CARTESIAN_POINT('Ctrl Pts',(-7.0987250270912,3.73918273690758,3.09050050603284));
#17221=CARTESIAN_POINT('Ctrl Pts',(-6.79624457301434,3.19090820274708,3.17383813798714));
#17222=CARTESIAN_POINT('Ctrl Pts',(-6.24569553319637,2.88613001714052,3.25758997671661));
#17223=CARTESIAN_POINT('Ctrl Pts',(-5.61454866908592,2.92117214212433,3.34171971865797));
#17224=CARTESIAN_POINT('Ctrl Pts',(-5.09672508083302,3.28814927637395,3.4261891931306));
#17225=CARTESIAN_POINT('Ctrl Pts',(-4.8527010496301,3.87647815686147,3.51095811781651));
#17226=CARTESIAN_POINT('Ctrl Pts',(-4.95944840393067,4.50636398239007,3.595984371598));
#17227=CARTESIAN_POINT('Ctrl Pts',(-5.38609475348018,4.98408471257233,3.68122458091311));
#17228=CARTESIAN_POINT('Ctrl Pts',(-6.00268079420748,5.16189327329318,3.76663345374862));
#17229=CARTESIAN_POINT('Ctrl Pts',(-6.62039054353995,4.98411118093899,3.85216610920168));
#17230=CARTESIAN_POINT('Ctrl Pts',(-7.03296634594375,4.52220299265115,3.93460295352821));
#17231=CARTESIAN_POINT('Ctrl Pts',(-7.14985065007003,3.94288654783804,4.01389927783044));
#17232=CARTESIAN_POINT('Ctrl Pts',(-6.98272205096131,3.40093752568897,4.0900113004944));
#17233=CARTESIAN_POINT('Ctrl Pts',(-6.57680875018895,3.00520046094579,4.16608365584876));
#17234=CARTESIAN_POINT('Ctrl Pts',(-6.03173171378752,2.85157669802245,4.24208403850743));
#17235=CARTESIAN_POINT('Ctrl Pts',(-5.48034738502237,2.97784080438086,4.31797832595391));
#17236=CARTESIAN_POINT('Ctrl Pts',(-5.09268849546396,3.32036229583066,4.3874112267225));
#17237=CARTESIAN_POINT('Ctrl Pts',(-4.90777324710137,3.74504999230099,4.45041329672765));
#17238=CARTESIAN_POINT('Ctrl Pts',(-4.89217896507905,4.16075012922992,4.50700493335702));
#17239=CARTESIAN_POINT('Ctrl Pts',(-5.02947267525229,4.55245617462658,4.56347581988345));
#17240=CARTESIAN_POINT('Ctrl Pts',(-5.32947452049713,4.90147627896693,4.62607044249519));
#17241=CARTESIAN_POINT('Ctrl Pts',(-5.79584535398848,5.11161943763673,4.69471754610501));
#17242=CARTESIAN_POINT('Ctrl Pts',(-6.35014451448374,5.06959102637412,4.7693250241412));
#17243=CARTESIAN_POINT('Ctrl Pts',(-6.77631798822209,4.79395495836344,4.83741703394908));
#17244=CARTESIAN_POINT('Ctrl Pts',(-7.01666455556856,4.40998698374066,4.89908002516321));
#17245=CARTESIAN_POINT('Ctrl Pts',(-7.11887670267137,3.87728204193206,4.97281129786051));
#17246=CARTESIAN_POINT('Ctrl Pts',(-6.85969875513886,3.21712465631829,5.06443234656144));
#17247=CARTESIAN_POINT('Ctrl Pts',(-6.09709548778395,2.85143338377357,5.17348766082218));
#17248=CARTESIAN_POINT('Ctrl Pts',(-5.29731395843599,3.09982709410499,5.28157901580182));
#17249=CARTESIAN_POINT('Ctrl Pts',(-4.88367792874778,3.81923523883344,5.38866556777043));
#17250=CARTESIAN_POINT('Ctrl Pts',(-5.06792313288877,4.61994565311358,5.49470491264318));
#17251=CARTESIAN_POINT('Ctrl Pts',(-5.74134532638002,5.07694585878306,5.59967630177535));
#17252=CARTESIAN_POINT('Ctrl Pts',(-6.35946722683167,4.98198830174697,5.68046971855626));
#17253=CARTESIAN_POINT('Ctrl Pts',(-6.69137247180265,4.72895391359148,5.7377846585707));
#17254=CARTESIAN_POINT('Ctrl Pts',(-6.89903102024635,4.46928826285102,5.78347589255367));
#17255=CARTESIAN_POINT('Ctrl Pts',(-7.02364136198497,4.06457023003713,5.84028303985189));
#17256=CARTESIAN_POINT('Ctrl Pts',(-6.92300892708766,3.5704067168229,5.90797894643917));
#17257=CARTESIAN_POINT('Ctrl Pts',(-6.60082158074705,3.18688178295313,5.97519979799271));
#17258=CARTESIAN_POINT('Ctrl Pts',(-6.13768958587062,3.00572129709394,6.04195922782834));
#17259=CARTESIAN_POINT('Ctrl Pts',(-5.6883298773806,3.06253696090835,6.10274000217679));
#17260=CARTESIAN_POINT('Ctrl Pts',(-5.34722099251186,3.27774259824664,6.15767505319115));
#17261=CARTESIAN_POINT('Ctrl Pts',(-5.0596350596403,3.66561735956058,6.22327451214416));
#17262=CARTESIAN_POINT('Ctrl Pts',(-5.02173651226817,4.16716900833336,6.28840828372746));
#17263=CARTESIAN_POINT('Ctrl Pts',(-5.24614992976449,4.58745247284312,6.35310163465723));
#17264=CARTESIAN_POINT('Ctrl Pts',(-5.51477848997985,4.81896891835744,6.40141121346934));
#17265=CARTESIAN_POINT('Ctrl Pts',(-5.84881374774272,4.9354787272431,6.4495201665249));
#17266=CARTESIAN_POINT('Ctrl Pts',(-6.25943186378334,4.92033084311256,6.50542267537317));
#17267=CARTESIAN_POINT('Ctrl Pts',(-6.67740663203018,4.68935725087564,6.56901532400741));
#17268=CARTESIAN_POINT('Ctrl Pts',(-6.93578121619537,4.22100070878716,6.64018116904655));
#17269=CARTESIAN_POINT('Ctrl Pts',(-6.9104300619441,3.77859534030824,6.699213603944));
#17270=CARTESIAN_POINT('Ctrl Pts',(-6.75240590109235,3.47372741247044,6.74628509889055));
#17271=CARTESIAN_POINT('Ctrl Pts',(-6.55640934718448,3.26621135700427,6.78543648927768));
#17272=CARTESIAN_POINT('Ctrl Pts',(-6.27707437535794,3.11861349905881,6.82841657096604));
#17273=CARTESIAN_POINT('Ctrl Pts',(-5.9355022847588,3.08022875183803,6.87520052017041));
#17274=CARTESIAN_POINT('Ctrl Pts',(-5.54858200380153,3.1836250601501,6.92968354415467));
#17275=CARTESIAN_POINT('Ctrl Pts',(-5.20045972734387,3.49445659550131,6.99184374671821));
#17276=CARTESIAN_POINT('Ctrl Pts',(-5.05544732191987,3.99851041473827,7.06165119985256));
#17277=CARTESIAN_POINT('Ctrl Pts',(-5.20048107826059,4.50175960678276,7.13139174737956));
#17278=CARTESIAN_POINT('Ctrl Pts',(-5.59093790031351,4.85072254510397,7.20110862526653));
#17279=CARTESIAN_POINT('Ctrl Pts',(-6.10734774732503,4.93850031945277,7.27085082830924));
#17280=CARTESIAN_POINT('Ctrl Pts',(-6.59183509574101,4.7379341695227,7.34066464130002));
#17281=CARTESIAN_POINT('Ctrl Pts',(-6.89590284323148,4.30964148274272,7.41059704126021));
#17282=CARTESIAN_POINT('Ctrl Pts',(-6.92561924919337,3.78399509029939,7.48069377094016));
#17283=CARTESIAN_POINT('Ctrl Pts',(-6.6704002715619,3.32170621392155,7.5509998057238));
#17284=CARTESIAN_POINT('Ctrl Pts',(-6.20670653876933,3.06509997300355,7.62155879348131));
#17285=CARTESIAN_POINT('Ctrl Pts',(-5.67534724500118,3.09460421450561,7.69241293056779));
#17286=CARTESIAN_POINT('Ctrl Pts',(-5.23904547633351,3.40371059691615,7.76360262044568));
#17287=CARTESIAN_POINT('Ctrl Pts',(-5.0329663099472,3.90014632476456,7.83516634990396));
#17288=CARTESIAN_POINT('Ctrl Pts',(-5.12305877544344,4.43317697771956,7.90714029938048));
#17289=CARTESIAN_POINT('Ctrl Pts',(-5.48516295948042,4.83908746429057,7.97955849057881));
#17290=CARTESIAN_POINT('Ctrl Pts',(-6.01107465918283,4.99114822692247,8.05245176655152));
#17291=CARTESIAN_POINT('Ctrl Pts',(-6.54108875049124,4.83908239809763,8.1258494812478));
#17292=CARTESIAN_POINT('Ctrl Pts',(-6.89755173489568,4.44070311733813,8.19703730133364));
#17293=CARTESIAN_POINT('Ctrl Pts',(-6.99966563994677,3.93733853721186,8.26597111831699));
#17294=CARTESIAN_POINT('Ctrl Pts',(-6.8536012652616,3.46307615160578,8.33258743659512));
#17295=CARTESIAN_POINT('Ctrl Pts',(-6.52611138411337,3.14291249345024,8.39407543281095));
#17296=CARTESIAN_POINT('Ctrl Pts',(-6.13582853537318,3.00649193719368,8.45031886967759));
#17297=CARTESIAN_POINT('Ctrl Pts',(-5.76220105188843,3.02015704448408,8.50120517126138));
#17298=CARTESIAN_POINT('Ctrl Pts',(-5.41757335971822,3.17041692695101,8.55235642674854));
#17299=CARTESIAN_POINT('Ctrl Pts',(-5.15021641590212,3.43748811582643,8.60378222122026));
#17300=CARTESIAN_POINT('Ctrl Pts',(-4.99809986343188,3.78564552616636,8.65547998995423));
#17301=CARTESIAN_POINT('Ctrl Pts',(-4.98362774422425,4.16729388058725,8.70744993309881));
#17302=CARTESIAN_POINT('Ctrl Pts',(-5.11024697508206,4.52974174117404,8.75969162933513));
#17303=CARTESIAN_POINT('Ctrl Pts',(-5.36183465340263,4.82237913826861,8.81220383694267));
#17304=CARTESIAN_POINT('Ctrl Pts',(-5.70469256863376,5.00379700216032,8.86498466304636));
#17305=CARTESIAN_POINT('Ctrl Pts',(-6.09208369431142,5.04762573267528,8.91803146859742));
#17306=CARTESIAN_POINT('Ctrl Pts',(-6.47056983558372,4.94639948026783,8.97134097339838));
#17307=CARTESIAN_POINT('Ctrl Pts',(-6.78746858719032,4.71274045756303,9.02490910160121));
#17308=CARTESIAN_POINT('Ctrl Pts',(-6.99804433390308,4.37791298839973,9.07873133117115));
#17309=CARTESIAN_POINT('Ctrl Pts',(-7.07219332762122,3.98740319786627,9.13280196225214));
#17310=CARTESIAN_POINT('Ctrl Pts',(-6.99796865015276,3.59525453990437,9.18711581050414));
#17311=CARTESIAN_POINT('Ctrl Pts',(-6.76140078434104,3.2176912418475,9.24772569638974));
#17312=CARTESIAN_POINT('Ctrl Pts',(-6.34225949707073,2.94654602106377,9.31472311482269));
#17313=CARTESIAN_POINT('Ctrl Pts',(-5.79639322685134,2.90560751314568,9.3882003670644));
#17314=CARTESIAN_POINT('Ctrl Pts',(-5.27370444272467,3.14075473304909,9.46511866155133));
#17315=CARTESIAN_POINT('Ctrl Pts',(-4.92371803536237,3.63287013680252,9.54550949397408));
#17316=CARTESIAN_POINT('Ctrl Pts',(-4.88802166561496,4.26218457037089,9.62939471067557));
#17317=CARTESIAN_POINT('Ctrl Pts',(-5.19387931501792,4.81633827697949,9.71364499530948));
#17318=CARTESIAN_POINT('Ctrl Pts',(-5.74991952335929,5.12402428928409,9.79822162675657));
#17319=CARTESIAN_POINT('Ctrl Pts',(-6.38656191712891,5.0885391306891,9.88308361150577));
#17320=CARTESIAN_POINT('Ctrl Pts',(-6.90822667172928,4.71869213404092,9.96818846822383));
#17321=CARTESIAN_POINT('Ctrl Pts',(-7.15369278117839,4.12658524801911,10.0534921977017));
#17322=CARTESIAN_POINT('Ctrl Pts',(-7.04627827661993,3.49350501160261,10.1389496543118));
#17323=CARTESIAN_POINT('Ctrl Pts',(-6.61793136444462,3.0140348706312,10.2245147901346));
#17324=CARTESIAN_POINT('Ctrl Pts',(-5.99969047434799,2.83587138114131,10.3101409223404));
#17325=CARTESIAN_POINT('Ctrl Pts',(-5.38133414015581,3.01401924516413,10.3957810076217));
#17326=CARTESIAN_POINT('Ctrl Pts',(-4.95274187669847,3.49369758179628,10.481387897791));
#17327=CARTESIAN_POINT('Ctrl Pts',(-4.84520028211577,4.12729592446544,10.5669146789137));
#17328=CARTESIAN_POINT('Ctrl Pts',(-5.09092458014618,4.72009886759013,10.6523148677484));
#17329=CARTESIAN_POINT('Ctrl Pts',(-5.61335583694406,5.09051867229157,10.7375427577537));
#17330=CARTESIAN_POINT('Ctrl Pts',(-6.25117077894511,5.12607085917612,10.8225535720965));
#17331=CARTESIAN_POINT('Ctrl Pts',(-6.80841662056156,4.81774324430063,10.9073040023736));
#17332=CARTESIAN_POINT('Ctrl Pts',(-7.11508736240155,4.2621592301609,10.9917518238937));
#17333=CARTESIAN_POINT('Ctrl Pts',(-7.0792883317528,3.63115822330435,11.0758574987941));
#17334=CARTESIAN_POINT('Ctrl Pts',(-6.71491091945052,3.11823669279566,11.1595814344114));
#17335=CARTESIAN_POINT('Ctrl Pts',(-6.13641410951145,2.87910001310329,11.2428908007876));
#17336=CARTESIAN_POINT('Ctrl Pts',(-5.52273543986151,2.98368129161145,11.3257449331281));
#17337=CARTESIAN_POINT('Ctrl Pts',(-5.06157565192072,3.39673596202277,11.4081288381091));
#17338=CARTESIAN_POINT('Ctrl Pts',(-4.94849818871645,3.79037870846202,11.4626969504328));
#17339=CARTESIAN_POINT('Ctrl Pts',(-4.94847164137573,3.98757933453,11.4899208404099));
#17340=CARTESIAN_POINT('Ctrl Pts',(-5.00000184100681,4.0136754734751,2.60093950625076));
#17341=CARTESIAN_POINT('Ctrl Pts',(-5.00002711936209,4.20144961727963,2.62686205390075));
#17342=CARTESIAN_POINT('Ctrl Pts',(-5.1076914443916,4.57620101292901,2.67882571929646));
#17343=CARTESIAN_POINT('Ctrl Pts',(-5.54731085839696,4.97011855968613,2.75738770095752));
#17344=CARTESIAN_POINT('Ctrl Pts',(-6.13330829028169,5.07009398433603,2.83651804650349));
#17345=CARTESIAN_POINT('Ctrl Pts',(-6.68676060294283,4.84148936906199,2.91622569034364));
#17346=CARTESIAN_POINT('Ctrl Pts',(-7.03617542740839,4.34995411926946,2.99649057036664));
#17347=CARTESIAN_POINT('Ctrl Pts',(-7.07077171566156,3.74380977688242,3.07730075350998));
#17348=CARTESIAN_POINT('Ctrl Pts',(-6.77566001133407,3.20870450421941,3.15863603264667));
#17349=CARTESIAN_POINT('Ctrl Pts',(-6.23777975703619,2.91082274760045,3.24047540010177));
#17350=CARTESIAN_POINT('Ctrl Pts',(-5.62027751939497,2.94499359194798,3.32279385402167));
#17351=CARTESIAN_POINT('Ctrl Pts',(-5.1128578559771,3.30444603110391,3.40556404882598));
#17352=CARTESIAN_POINT('Ctrl Pts',(-4.87328209631149,3.88170381609706,3.48875576249667));
#17353=CARTESIAN_POINT('Ctrl Pts',(-4.97806047014568,4.50081578134862,3.57233636795591));
#17354=CARTESIAN_POINT('Ctrl Pts',(-5.39799694068156,4.97124635132397,3.65627091939543));
#17355=CARTESIAN_POINT('Ctrl Pts',(-6.00608186722498,5.1467635917961,3.7405223892875));
#17356=CARTESIAN_POINT('Ctrl Pts',(-6.61648592829516,4.97125245378467,3.82505187703477));
#17357=CARTESIAN_POINT('Ctrl Pts',(-7.02504723026834,4.51407458863333,3.90667930466183));
#17358=CARTESIAN_POINT('Ctrl Pts',(-7.14109507248108,3.93953170138583,3.98533819578826));
#17359=CARTESIAN_POINT('Ctrl Pts',(-6.97515546374893,3.40104443225745,4.06097495793453));
#17360=CARTESIAN_POINT('Ctrl Pts',(-6.57122653386479,3.00706128325563,4.13670514732847));
#17361=CARTESIAN_POINT('Ctrl Pts',(-6.02775857632327,2.85377271371871,4.21249751130402));
#17362=CARTESIAN_POINT('Ctrl Pts',(-5.47693199324532,2.97976879840739,4.28832050275612));
#17363=CARTESIAN_POINT('Ctrl Pts',(-5.08889329636147,3.32248782371839,4.35782394322737));
#17364=CARTESIAN_POINT('Ctrl Pts',(-4.90348334427995,3.74815768282725,4.42098503121462));
#17365=CARTESIAN_POINT('Ctrl Pts',(-4.88777846541416,4.16541417756998,4.47779829335302));
#17366=CARTESIAN_POINT('Ctrl Pts',(-5.02572337488508,4.5591407782775,4.53456660974454));
#17367=CARTESIAN_POINT('Ctrl Pts',(-5.32762081329308,4.91046292297288,4.59757802398128));
#17368=CARTESIAN_POINT('Ctrl Pts',(-5.79769987729577,5.12240617534609,4.6667893141555));
#17369=CARTESIAN_POINT('Ctrl Pts',(-6.35744977854988,5.0800953582818,4.74213609062164));
#17370=CARTESIAN_POINT('Ctrl Pts',(-6.7886388886812,4.80135715932747,4.81103357029135));
#17371=CARTESIAN_POINT('Ctrl Pts',(-7.03217914396847,4.41239214657722,4.87351124701705));
#17372=CARTESIAN_POINT('Ctrl Pts',(-7.13592863330475,3.87207852021905,4.94830807653976));
#17373=CARTESIAN_POINT('Ctrl Pts',(-6.87284718079957,3.20107467373212,5.04144479366485));
#17374=CARTESIAN_POINT('Ctrl Pts',(-6.09623481157017,2.82823992504595,5.15254762809713));
#17375=CARTESIAN_POINT('Ctrl Pts',(-5.27971004197149,3.08146490109176,5.26291010705797));
#17376=CARTESIAN_POINT('Ctrl Pts',(-4.85635349881296,3.81715131471987,5.37246078991772));
#17377=CARTESIAN_POINT('Ctrl Pts',(-5.04487949063783,4.63769677411038,5.48113679376609));
#17378=CARTESIAN_POINT('Ctrl Pts',(-5.73589746055469,5.10693196272956,5.58888446285182));
#17379=CARTESIAN_POINT('Ctrl Pts',(-6.37118793757295,5.00949360744693,5.67193196549858));
#17380=CARTESIAN_POINT('Ctrl Pts',(-6.71254361053678,4.74926813559046,5.73087908447486));
#17381=CARTESIAN_POINT('Ctrl Pts',(-6.92618421314144,4.48213635150675,5.77788659686335));
#17382=CARTESIAN_POINT('Ctrl Pts',(-7.05447791083229,4.06557532936466,5.83636209009091));
#17383=CARTESIAN_POINT('Ctrl Pts',(-6.95088091422359,3.55670409484484,5.90607316301112));
#17384=CARTESIAN_POINT('Ctrl Pts',(-6.61900788359635,3.16160526086392,5.97532164754671));
#17385=CARTESIAN_POINT('Ctrl Pts',(-6.14183402203666,2.97493714351951,6.0441065734333));
#17386=CARTESIAN_POINT('Ctrl Pts',(-5.67880942079896,3.03347123408109,6.10673564359386));
#17387=CARTESIAN_POINT('Ctrl Pts',(-5.32735160410172,3.25520230218429,6.16333652454754));
#17388=CARTESIAN_POINT('Ctrl Pts',(-5.03108251682038,3.65479384285351,6.23091649770626));
#17389=CARTESIAN_POINT('Ctrl Pts',(-4.99209121035488,4.17131828916311,6.29799027327816));
#17390=CARTESIAN_POINT('Ctrl Pts',(-5.22308647377139,4.60388582873653,6.36457330678434));
#17391=CARTESIAN_POINT('Ctrl Pts',(-5.49945070307415,4.84205518395227,6.4142703184249));
#17392=CARTESIAN_POINT('Ctrl Pts',(-5.8429108649416,4.96183684549319,6.46373244635463));
#17393=CARTESIAN_POINT('Ctrl Pts',(-6.26484181971828,4.94625056066266,6.52117144061682));
#17394=CARTESIAN_POINT('Ctrl Pts',(-6.69390577408147,4.70907736638303,6.58644589945804));
#17395=CARTESIAN_POINT('Ctrl Pts',(-6.95873462103172,4.22881797506906,6.65940509116432));
#17396=CARTESIAN_POINT('Ctrl Pts',(-6.93269246532923,3.77588585116234,6.71983222414211));
#17397=CARTESIAN_POINT('Ctrl Pts',(-6.77107468324783,3.46412923688142,6.7679659145118));
#17398=CARTESIAN_POINT('Ctrl Pts',(-6.57079871082626,3.25210408080074,6.80796630929164));
#17399=CARTESIAN_POINT('Ctrl Pts',(-6.28566327773964,3.10148204150563,6.85183024182226));
#17400=CARTESIAN_POINT('Ctrl Pts',(-5.9374350403567,3.06238692304077,6.89952195896654));
#17401=CARTESIAN_POINT('Ctrl Pts',(-5.54350254185785,3.16770824417749,6.95498839067594));
#17402=CARTESIAN_POINT('Ctrl Pts',(-5.18977130243312,3.48372162057587,7.01814871426604));
#17403=CARTESIAN_POINT('Ctrl Pts',(-5.04285761799324,3.99497433346206,7.0889328817521));
#17404=CARTESIAN_POINT('Ctrl Pts',(-5.18978309684873,4.50416337482064,7.15948666242575));
#17405=CARTESIAN_POINT('Ctrl Pts',(-5.58408091231752,4.85632154197909,7.22985222665258));
#17406=CARTESIAN_POINT('Ctrl Pts',(-6.10418851591415,4.94454356395432,7.30007283487924));
#17407=CARTESIAN_POINT('Ctrl Pts',(-6.59084588507658,4.74288104801731,7.37019262264957));
#17408=CARTESIAN_POINT('Ctrl Pts',(-6.89540829263521,4.31357351131412,7.44025632549589));
#17409=CARTESIAN_POINT('Ctrl Pts',(-6.92492923689232,3.78812028153619,7.51030900574892));
#17410=CARTESIAN_POINT('Ctrl Pts',(-6.67028427013333,3.32725098620657,7.58039577698737));
#17411=CARTESIAN_POINT('Ctrl Pts',(-6.20897623341015,3.0721729365591,7.65056157443552));
#17412=CARTESIAN_POINT('Ctrl Pts',(-5.68173783558839,3.10162769981329,7.72085085716389));
#17413=CARTESIAN_POINT('Ctrl Pts',(-5.24992919279951,3.40776503869049,7.79130734597953));
#17414=CARTESIAN_POINT('Ctrl Pts',(-5.0465424843122,3.89815513625059,7.86197377424775));
#17415=CARTESIAN_POINT('Ctrl Pts',(-5.13549244911485,4.42345796985394,7.9328916443029));
#17416=CARTESIAN_POINT('Ctrl Pts',(-5.49174629490197,4.82258141736487,8.00410096577713));
#17417=CARTESIAN_POINT('Ctrl Pts',(-6.00803868168598,4.97171279548103,8.07564000534741));
#17418=CARTESIAN_POINT('Ctrl Pts',(-6.52735154266829,4.82257974695955,8.1475451059773));
#17419=CARTESIAN_POINT('Ctrl Pts',(-6.87597910605558,4.43277936154282,8.2171724616343));
#17420=CARTESIAN_POINT('Ctrl Pts',(-6.97565473561711,3.94102818366579,8.28449961898768));
#17421=CARTESIAN_POINT('Ctrl Pts',(-6.8330580514463,3.47827883486752,8.34949563910535));
#17422=CARTESIAN_POINT('Ctrl Pts',(-6.51380412257741,3.1662390255362,8.40942447363317));
#17423=CARTESIAN_POINT('Ctrl Pts',(-6.13368043091516,3.03340218960474,8.46419547601407));
#17424=CARTESIAN_POINT('Ctrl Pts',(-5.77000963425156,3.04672415558585,8.51371979129401));
#17425=CARTESIAN_POINT('Ctrl Pts',(-5.43474033823938,3.19292650787483,8.56348049163152));
#17426=CARTESIAN_POINT('Ctrl Pts',(-5.17477216956946,3.45264130135924,8.61348288970698));
#17427=CARTESIAN_POINT('Ctrl Pts',(-5.02692180394174,3.79107624660051,8.6637316830418));
#17428=CARTESIAN_POINT('Ctrl Pts',(-5.012872576251,4.16195256384123,8.7142309145088));
#17429=CARTESIAN_POINT('Ctrl Pts',(-5.13590369868626,4.51409239039593,8.76498396821864));
#17430=CARTESIAN_POINT('Ctrl Pts',(-5.38031427946466,4.79836661872066,8.81599356007185));
#17431=CARTESIAN_POINT('Ctrl Pts',(-5.71336668770006,4.97458793379134,8.86726173279411));
#17432=CARTESIAN_POINT('Ctrl Pts',(-6.08968356313292,5.01715924274108,8.918789847283));
#17433=CARTESIAN_POINT('Ctrl Pts',(-6.45738481100365,4.91881570416212,8.9705785818587));
#17434=CARTESIAN_POINT('Ctrl Pts',(-6.76530671813857,4.69177684003305,9.02262792715958));
#17435=CARTESIAN_POINT('Ctrl Pts',(-6.96997065785482,4.36635789720065,9.07493719271063));
#17436=CARTESIAN_POINT('Ctrl Pts',(-7.04206467317586,3.98670152421777,9.12750499448518));
#17437=CARTESIAN_POINT('Ctrl Pts',(-6.96988775131722,3.60530323601265,9.18032928987629));
#17438=CARTESIAN_POINT('Ctrl Pts',(-6.7397150976367,3.23792225540337,9.23930487839808));
#17439=CARTESIAN_POINT('Ctrl Pts',(-6.33166237507248,2.97390330552954,9.30453505300732));
#17440=CARTESIAN_POINT('Ctrl Pts',(-5.79979171434613,2.93396143628525,9.37613052323128));
#17441=CARTESIAN_POINT('Ctrl Pts',(-5.29001663621426,3.16323503239153,9.45115011122364));
#17442=CARTESIAN_POINT('Ctrl Pts',(-4.94825545210904,3.64363042187255,9.52964181259955));
#17443=CARTESIAN_POINT('Ctrl Pts',(-4.91325516498484,4.25878443889604,9.61164803507556));
#17444=CARTESIAN_POINT('Ctrl Pts',(-5.2125378502354,4.80126773521892,9.69412424268727));
#17445=CARTESIAN_POINT('Ctrl Pts',(-5.75754644935023,5.10299443985526,9.77704205666351));
#17446=CARTESIAN_POINT('Ctrl Pts',(-6.38261067907029,5.06829058753974,9.86037045595682));
#17447=CARTESIAN_POINT('Ctrl Pts',(-6.89571009340608,4.70469230712254,9.94407602284259));
#17448=CARTESIAN_POINT('Ctrl Pts',(-7.13766387710299,4.12145232028498,10.0281230888647));
#17449=CARTESIAN_POINT('Ctrl Pts',(-7.03181245317105,3.49664097659948,10.112473958668));
#17450=CARTESIAN_POINT('Ctrl Pts',(-6.60841264630813,3.02246212675956,10.1970891533592));
#17451=CARTESIAN_POINT('Ctrl Pts',(-5.99601006835875,2.8458044826624,10.2819276244449));
#17452=CARTESIAN_POINT('Ctrl Pts',(-5.38219522105592,3.02246199100347,10.3669470032346));
#17453=CARTESIAN_POINT('Ctrl Pts',(-4.95579995827654,3.49941222674329,10.452103831618));
#17454=CARTESIAN_POINT('Ctrl Pts',(-4.84844583817861,4.13081136700949,10.5373538681711));
#17455=CARTESIAN_POINT('Ctrl Pts',(-5.0936581339001,4.72286468788687,10.6226522983686));
#17456=CARTESIAN_POINT('Ctrl Pts',(-5.61632959368519,5.09368411438882,10.7079540155997));
#17457=CARTESIAN_POINT('Ctrl Pts',(-6.25587144748665,5.12951914158568,10.7932138961696));
#17458=CARTESIAN_POINT('Ctrl Pts',(-6.81586867421465,4.81987787722662,10.8783870694892));
#17459=CARTESIAN_POINT('Ctrl Pts',(-7.12478685219004,4.26058878480156,10.9634291596385));
#17460=CARTESIAN_POINT('Ctrl Pts',(-7.08884111245123,3.62399110135786,11.0482965343607));
#17461=CARTESIAN_POINT('Ctrl Pts',(-6.72064073263906,3.10540887765364,11.132946666915));
#17462=CARTESIAN_POINT('Ctrl Pts',(-6.13478909423228,2.86304904084892,11.2173381176655));
#17463=CARTESIAN_POINT('Ctrl Pts',(-5.51202996456676,2.96902046658306,11.3014313460436));
#17464=CARTESIAN_POINT('Ctrl Pts',(-5.04310782052529,3.38875866553956,11.3851878225675));
#17465=CARTESIAN_POINT('Ctrl Pts',(-4.92780437314741,3.78964966219835,11.4407823887586));
#17466=CARTESIAN_POINT('Ctrl Pts',(-4.9277773302074,3.99053173009658,11.468514508194));
#17467=CARTESIAN_POINT('',(-5.00000184100681,4.0136754734751,2.60093950625076));
#17468=CARTESIAN_POINT('Origin',(-5.,4.,2.7));
#17469=CARTESIAN_POINT('',(-4.9277773302074,3.99053173009658,11.468514508194));
#17470=CARTESIAN_POINT('Ctrl Pts',(-5.00000184100681,4.0136754734751,2.60093950625076));
#17471=CARTESIAN_POINT('Ctrl Pts',(-5.00002711936209,4.20144961727963,2.62686205390075));
#17472=CARTESIAN_POINT('Ctrl Pts',(-5.1076914443916,4.57620101292901,2.67882571929646));
#17473=CARTESIAN_POINT('Ctrl Pts',(-5.54731085839696,4.97011855968613,2.75738770095752));
#17474=CARTESIAN_POINT('Ctrl Pts',(-6.13330829028169,5.07009398433603,2.83651804650349));
#17475=CARTESIAN_POINT('Ctrl Pts',(-6.68676060294283,4.84148936906199,2.91622569034364));
#17476=CARTESIAN_POINT('Ctrl Pts',(-7.03617542740839,4.34995411926946,2.99649057036664));
#17477=CARTESIAN_POINT('Ctrl Pts',(-7.07077171566156,3.74380977688242,3.07730075350998));
#17478=CARTESIAN_POINT('Ctrl Pts',(-6.77566001133407,3.20870450421941,3.15863603264667));
#17479=CARTESIAN_POINT('Ctrl Pts',(-6.23777975703619,2.91082274760045,3.24047540010177));
#17480=CARTESIAN_POINT('Ctrl Pts',(-5.62027751939497,2.94499359194798,3.32279385402167));
#17481=CARTESIAN_POINT('Ctrl Pts',(-5.1128578559771,3.30444603110391,3.40556404882598));
#17482=CARTESIAN_POINT('Ctrl Pts',(-4.87328209631149,3.88170381609706,3.48875576249667));
#17483=CARTESIAN_POINT('Ctrl Pts',(-4.97806047014568,4.50081578134862,3.57233636795591));
#17484=CARTESIAN_POINT('Ctrl Pts',(-5.39799694068156,4.97124635132397,3.65627091939543));
#17485=CARTESIAN_POINT('Ctrl Pts',(-6.00608186722498,5.1467635917961,3.7405223892875));
#17486=CARTESIAN_POINT('Ctrl Pts',(-6.61648592829516,4.97125245378467,3.82505187703477));
#17487=CARTESIAN_POINT('Ctrl Pts',(-7.02504723026834,4.51407458863333,3.90667930466183));
#17488=CARTESIAN_POINT('Ctrl Pts',(-7.14109507248108,3.93953170138583,3.98533819578826));
#17489=CARTESIAN_POINT('Ctrl Pts',(-6.97515546374893,3.40104443225745,4.06097495793453));
#17490=CARTESIAN_POINT('Ctrl Pts',(-6.57122653386479,3.00706128325563,4.13670514732847));
#17491=CARTESIAN_POINT('Ctrl Pts',(-6.02775857632327,2.85377271371871,4.21249751130402));
#17492=CARTESIAN_POINT('Ctrl Pts',(-5.47693199324532,2.97976879840739,4.28832050275612));
#17493=CARTESIAN_POINT('Ctrl Pts',(-5.08889329636147,3.32248782371839,4.35782394322737));
#17494=CARTESIAN_POINT('Ctrl Pts',(-4.90348334427995,3.74815768282725,4.42098503121462));
#17495=CARTESIAN_POINT('Ctrl Pts',(-4.88777846541416,4.16541417756998,4.47779829335302));
#17496=CARTESIAN_POINT('Ctrl Pts',(-5.02572337488508,4.5591407782775,4.53456660974454));
#17497=CARTESIAN_POINT('Ctrl Pts',(-5.32762081329308,4.91046292297288,4.59757802398128));
#17498=CARTESIAN_POINT('Ctrl Pts',(-5.79769987729577,5.12240617534609,4.6667893141555));
#17499=CARTESIAN_POINT('Ctrl Pts',(-6.35744977854988,5.0800953582818,4.74213609062164));
#17500=CARTESIAN_POINT('Ctrl Pts',(-6.7886388886812,4.80135715932747,4.81103357029135));
#17501=CARTESIAN_POINT('Ctrl Pts',(-7.03217914396847,4.41239214657722,4.87351124701705));
#17502=CARTESIAN_POINT('Ctrl Pts',(-7.13592863330475,3.87207852021905,4.94830807653976));
#17503=CARTESIAN_POINT('Ctrl Pts',(-6.87284718079957,3.20107467373212,5.04144479366485));
#17504=CARTESIAN_POINT('Ctrl Pts',(-6.09623481157017,2.82823992504595,5.15254762809713));
#17505=CARTESIAN_POINT('Ctrl Pts',(-5.27971004197149,3.08146490109176,5.26291010705797));
#17506=CARTESIAN_POINT('Ctrl Pts',(-4.85635349881296,3.81715131471987,5.37246078991772));
#17507=CARTESIAN_POINT('Ctrl Pts',(-5.04487949063783,4.63769677411038,5.48113679376609));
#17508=CARTESIAN_POINT('Ctrl Pts',(-5.73589746055469,5.10693196272956,5.58888446285182));
#17509=CARTESIAN_POINT('Ctrl Pts',(-6.37118793757295,5.00949360744693,5.67193196549858));
#17510=CARTESIAN_POINT('Ctrl Pts',(-6.71254361053678,4.74926813559046,5.73087908447486));
#17511=CARTESIAN_POINT('Ctrl Pts',(-6.92618421314144,4.48213635150675,5.77788659686335));
#17512=CARTESIAN_POINT('Ctrl Pts',(-7.05447791083229,4.06557532936466,5.83636209009091));
#17513=CARTESIAN_POINT('Ctrl Pts',(-6.95088091422359,3.55670409484484,5.90607316301112));
#17514=CARTESIAN_POINT('Ctrl Pts',(-6.61900788359635,3.16160526086392,5.97532164754671));
#17515=CARTESIAN_POINT('Ctrl Pts',(-6.14183402203666,2.97493714351951,6.0441065734333));
#17516=CARTESIAN_POINT('Ctrl Pts',(-5.67880942079896,3.03347123408109,6.10673564359386));
#17517=CARTESIAN_POINT('Ctrl Pts',(-5.32735160410172,3.25520230218429,6.16333652454754));
#17518=CARTESIAN_POINT('Ctrl Pts',(-5.03108251682038,3.65479384285351,6.23091649770626));
#17519=CARTESIAN_POINT('Ctrl Pts',(-4.99209121035488,4.17131828916311,6.29799027327816));
#17520=CARTESIAN_POINT('Ctrl Pts',(-5.22308647377139,4.60388582873653,6.36457330678434));
#17521=CARTESIAN_POINT('Ctrl Pts',(-5.49945070307415,4.84205518395227,6.4142703184249));
#17522=CARTESIAN_POINT('Ctrl Pts',(-5.8429108649416,4.96183684549319,6.46373244635463));
#17523=CARTESIAN_POINT('Ctrl Pts',(-6.26484181971828,4.94625056066266,6.52117144061682));
#17524=CARTESIAN_POINT('Ctrl Pts',(-6.69390577408147,4.70907736638303,6.58644589945804));
#17525=CARTESIAN_POINT('Ctrl Pts',(-6.95873462103172,4.22881797506906,6.65940509116432));
#17526=CARTESIAN_POINT('Ctrl Pts',(-6.93269246532923,3.77588585116234,6.71983222414211));
#17527=CARTESIAN_POINT('Ctrl Pts',(-6.77107468324783,3.46412923688142,6.7679659145118));
#17528=CARTESIAN_POINT('Ctrl Pts',(-6.57079871082626,3.25210408080074,6.80796630929164));
#17529=CARTESIAN_POINT('Ctrl Pts',(-6.28566327773964,3.10148204150563,6.85183024182226));
#17530=CARTESIAN_POINT('Ctrl Pts',(-5.9374350403567,3.06238692304077,6.89952195896654));
#17531=CARTESIAN_POINT('Ctrl Pts',(-5.54350254185785,3.16770824417749,6.95498839067594));
#17532=CARTESIAN_POINT('Ctrl Pts',(-5.18977130243312,3.48372162057587,7.01814871426604));
#17533=CARTESIAN_POINT('Ctrl Pts',(-5.04285761799324,3.99497433346206,7.0889328817521));
#17534=CARTESIAN_POINT('Ctrl Pts',(-5.18978309684873,4.50416337482064,7.15948666242575));
#17535=CARTESIAN_POINT('Ctrl Pts',(-5.58408091231752,4.85632154197909,7.22985222665258));
#17536=CARTESIAN_POINT('Ctrl Pts',(-6.10418851591415,4.94454356395432,7.30007283487924));
#17537=CARTESIAN_POINT('Ctrl Pts',(-6.59084588507658,4.74288104801731,7.37019262264957));
#17538=CARTESIAN_POINT('Ctrl Pts',(-6.89540829263521,4.31357351131412,7.44025632549589));
#17539=CARTESIAN_POINT('Ctrl Pts',(-6.92492923689232,3.78812028153619,7.51030900574892));
#17540=CARTESIAN_POINT('Ctrl Pts',(-6.67028427013333,3.32725098620657,7.58039577698737));
#17541=CARTESIAN_POINT('Ctrl Pts',(-6.20897623341015,3.0721729365591,7.65056157443552));
#17542=CARTESIAN_POINT('Ctrl Pts',(-5.68173783558839,3.10162769981329,7.72085085716389));
#17543=CARTESIAN_POINT('Ctrl Pts',(-5.24992919279951,3.40776503869049,7.79130734597953));
#17544=CARTESIAN_POINT('Ctrl Pts',(-5.0465424843122,3.89815513625059,7.86197377424775));
#17545=CARTESIAN_POINT('Ctrl Pts',(-5.13549244911485,4.42345796985394,7.9328916443029));
#17546=CARTESIAN_POINT('Ctrl Pts',(-5.49174629490197,4.82258141736487,8.00410096577713));
#17547=CARTESIAN_POINT('Ctrl Pts',(-6.00803868168598,4.97171279548103,8.07564000534741));
#17548=CARTESIAN_POINT('Ctrl Pts',(-6.52735154266829,4.82257974695955,8.1475451059773));
#17549=CARTESIAN_POINT('Ctrl Pts',(-6.87597910605558,4.43277936154282,8.2171724616343));
#17550=CARTESIAN_POINT('Ctrl Pts',(-6.97565473561711,3.94102818366579,8.28449961898768));
#17551=CARTESIAN_POINT('Ctrl Pts',(-6.8330580514463,3.47827883486752,8.34949563910535));
#17552=CARTESIAN_POINT('Ctrl Pts',(-6.51380412257741,3.1662390255362,8.40942447363317));
#17553=CARTESIAN_POINT('Ctrl Pts',(-6.13368043091516,3.03340218960474,8.46419547601407));
#17554=CARTESIAN_POINT('Ctrl Pts',(-5.77000963425156,3.04672415558585,8.51371979129401));
#17555=CARTESIAN_POINT('Ctrl Pts',(-5.43474033823938,3.19292650787483,8.56348049163152));
#17556=CARTESIAN_POINT('Ctrl Pts',(-5.17477216956946,3.45264130135924,8.61348288970698));
#17557=CARTESIAN_POINT('Ctrl Pts',(-5.02692180394174,3.79107624660051,8.6637316830418));
#17558=CARTESIAN_POINT('Ctrl Pts',(-5.012872576251,4.16195256384123,8.7142309145088));
#17559=CARTESIAN_POINT('Ctrl Pts',(-5.13590369868626,4.51409239039593,8.76498396821864));
#17560=CARTESIAN_POINT('Ctrl Pts',(-5.38031427946466,4.79836661872066,8.81599356007185));
#17561=CARTESIAN_POINT('Ctrl Pts',(-5.71336668770006,4.97458793379134,8.86726173279411));
#17562=CARTESIAN_POINT('Ctrl Pts',(-6.08968356313292,5.01715924274108,8.918789847283));
#17563=CARTESIAN_POINT('Ctrl Pts',(-6.45738481100365,4.91881570416212,8.9705785818587));
#17564=CARTESIAN_POINT('Ctrl Pts',(-6.76530671813857,4.69177684003305,9.02262792715958));
#17565=CARTESIAN_POINT('Ctrl Pts',(-6.96997065785482,4.36635789720065,9.07493719271063));
#17566=CARTESIAN_POINT('Ctrl Pts',(-7.04206467317586,3.98670152421777,9.12750499448518));
#17567=CARTESIAN_POINT('Ctrl Pts',(-6.96988775131722,3.60530323601265,9.18032928987629));
#17568=CARTESIAN_POINT('Ctrl Pts',(-6.7397150976367,3.23792225540337,9.23930487839808));
#17569=CARTESIAN_POINT('Ctrl Pts',(-6.33166237507248,2.97390330552954,9.30453505300732));
#17570=CARTESIAN_POINT('Ctrl Pts',(-5.79979171434613,2.93396143628525,9.37613052323128));
#17571=CARTESIAN_POINT('Ctrl Pts',(-5.29001663621426,3.16323503239153,9.45115011122364));
#17572=CARTESIAN_POINT('Ctrl Pts',(-4.94825545210904,3.64363042187255,9.52964181259955));
#17573=CARTESIAN_POINT('Ctrl Pts',(-4.91325516498484,4.25878443889604,9.61164803507556));
#17574=CARTESIAN_POINT('Ctrl Pts',(-5.2125378502354,4.80126773521892,9.69412424268727));
#17575=CARTESIAN_POINT('Ctrl Pts',(-5.75754644935023,5.10299443985526,9.77704205666351));
#17576=CARTESIAN_POINT('Ctrl Pts',(-6.38261067907029,5.06829058753974,9.86037045595682));
#17577=CARTESIAN_POINT('Ctrl Pts',(-6.89571009340608,4.70469230712254,9.94407602284259));
#17578=CARTESIAN_POINT('Ctrl Pts',(-7.13766387710299,4.12145232028498,10.0281230888647));
#17579=CARTESIAN_POINT('Ctrl Pts',(-7.03181245317105,3.49664097659948,10.112473958668));
#17580=CARTESIAN_POINT('Ctrl Pts',(-6.60841264630813,3.02246212675956,10.1970891533592));
#17581=CARTESIAN_POINT('Ctrl Pts',(-5.99601006835875,2.8458044826624,10.2819276244449));
#17582=CARTESIAN_POINT('Ctrl Pts',(-5.38219522105592,3.02246199100347,10.3669470032346));
#17583=CARTESIAN_POINT('Ctrl Pts',(-4.95579995827654,3.49941222674329,10.452103831618));
#17584=CARTESIAN_POINT('Ctrl Pts',(-4.84844583817861,4.13081136700949,10.5373538681711));
#17585=CARTESIAN_POINT('Ctrl Pts',(-5.0936581339001,4.72286468788687,10.6226522983686));
#17586=CARTESIAN_POINT('Ctrl Pts',(-5.61632959368519,5.09368411438882,10.7079540155997));
#17587=CARTESIAN_POINT('Ctrl Pts',(-6.25587144748665,5.12951914158568,10.7932138961696));
#17588=CARTESIAN_POINT('Ctrl Pts',(-6.81586867421465,4.81987787722662,10.8783870694892));
#17589=CARTESIAN_POINT('Ctrl Pts',(-7.12478685219004,4.26058878480156,10.9634291596385));
#17590=CARTESIAN_POINT('Ctrl Pts',(-7.08884111245123,3.62399110135786,11.0482965343607));
#17591=CARTESIAN_POINT('Ctrl Pts',(-6.72064073263906,3.10540887765364,11.132946666915));
#17592=CARTESIAN_POINT('Ctrl Pts',(-6.13478909423228,2.86304904084892,11.2173381176655));
#17593=CARTESIAN_POINT('Ctrl Pts',(-5.51202996456676,2.96902046658306,11.3014313460436));
#17594=CARTESIAN_POINT('Ctrl Pts',(-5.04310782052529,3.38875866553956,11.3851878225675));
#17595=CARTESIAN_POINT('Ctrl Pts',(-4.92780437314741,3.78964966219835,11.4407823887586));
#17596=CARTESIAN_POINT('Ctrl Pts',(-4.9277773302074,3.99053173009658,11.468514508194));
#17597=CARTESIAN_POINT('Origin',(-5.,4.,11.4));
#17598=CARTESIAN_POINT('Origin',(-5.,4.,11.4));
#17599=CARTESIAN_POINT('Origin',(-5.,4.,2.7));
#22308=UNCERTAINTY_MEASURE_WITH_UNIT(LENGTH_MEASURE(0.001),#22395,
'DISTANCE_ACCURACY_VALUE',
'Maximum model space distance between geometric entities at asserted c
onnectivities');
#22343=UNCERTAINTY_MEASURE_WITH_UNIT(LENGTH_MEASURE(0.001),#22395,
'DISTANCE_ACCURACY_VALUE',
'Maximum model space distance between geometric entities at asserted c
onnectivities');
#22359=(
GEOMETRIC_REPRESENTATION_CONTEXT(3)
GLOBAL_UNCERTAINTY_ASSIGNED_CONTEXT((#22308))
GLOBAL_UNIT_ASSIGNED_CONTEXT((#22395,#22397,#22398))
REPRESENTATION_CONTEXT('','3D')
);
#22394=(
GEOMETRIC_REPRESENTATION_CONTEXT(3)
GLOBAL_UNCERTAINTY_ASSIGNED_CONTEXT((#22343))
GLOBAL_UNIT_ASSIGNED_CONTEXT((#22395,#22397,#22398))
REPRESENTATION_CONTEXT('','3D')
);
#22395=(
LENGTH_UNIT()
NAMED_UNIT(*)
SI_UNIT(.CENTI.,.METRE.)
);
#22397=(
NAMED_UNIT(*)
PLANE_ANGLE_UNIT()
SI_UNIT($,.RADIAN.)
);
#22398=(
NAMED_UNIT(*)
SI_UNIT($,.STERADIAN.)
SOLID_ANGLE_UNIT()
);
#22414=SHAPE_DEFINITION_REPRESENTATION(#22464,#22653);
#22464=PRODUCT_DEFINITION_SHAPE('',$,#22704);
#22653=SHAPE_REPRESENTATION('',(#10075),#22359);
#22688=PRODUCT_DEFINITION_CONTEXT('part definition',#22840,'design');
#22704=PRODUCT_DEFINITION('Installed compression spring (1)',
'Installed compression spring (1)',#22754,#22688);
#22754=PRODUCT_DEFINITION_FORMATION('',$,#22857);
#22840=APPLICATION_CONTEXT(
'Core Data for Automotive Mechanical Design Process');
#22841=PRODUCT_CONTEXT('part definition',#22840,'mechanical');
#22857=PRODUCT('Installed compression spring (1)',
'Installed compression spring (1)','Installed compression spring (1)',(#22841));
#22955=COLOUR_RGB('Grey',0.48,0.52,0.57);
#22956=FILL_AREA_STYLE_COLOUR('',#22955);
#22957=FILL_AREA_STYLE('',(#22956));
#22958=SURFACE_STYLE_FILL_AREA(#22957);
#22959=SURFACE_SIDE_STYLE('',(#22958));
#22960=SURFACE_STYLE_USAGE(.BOTH.,#22959);
#22961=PRESENTATION_STYLE_ASSIGNMENT((#22960));
ENDSEC;
END-ISO-10303-21;
